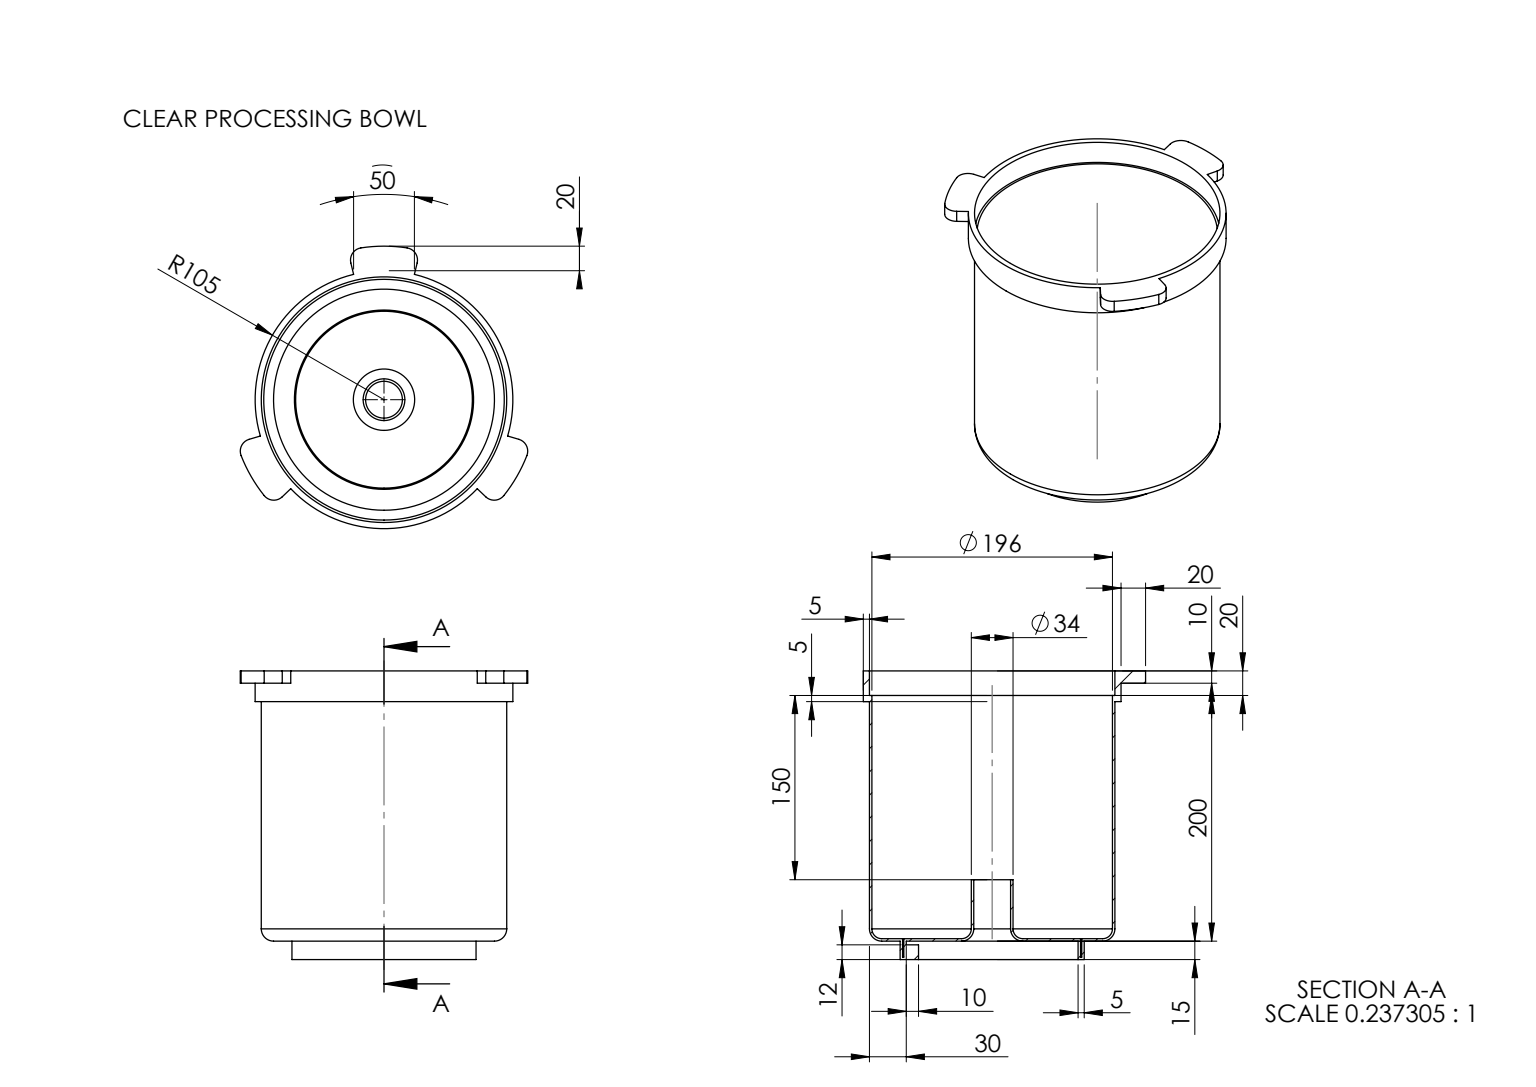
ISO-10303-21;
HEADER;
FILE_DESCRIPTION (('STEP AP214'),
    '1' );
FILE_NAME ('Clear Processing Bowl.step',
    '2026-10-08T14:59:03',
    ( '' ),
    ( '' ),
    'SwSTEP 2.0',
    'SolidWorks 2026',
    '' );
FILE_SCHEMA (( 'AUTOMOTIVE_DESIGN' ));
ENDSEC;

DATA;
#4=ORIENTED_EDGE ( 'NONE', *, *, #10707, .F. ) ;
#7=AXIS2_PLACEMENT_3D ( 'NONE', #9543, #8426, #7563 ) ;
#29=FACE_OUTER_BOUND ( 'NONE', #6935, .T. ) ;
#32=SURFACE_STYLE_FILL_AREA ( #12272 ) ;
#33=CARTESIAN_POINT ( 'NONE',  ( 0.000000000000000000, 62.00000000000000000, 0.000000000000000000 ) ) ;
#38=FACE_BOUND ( 'NONE', #4194, .T. ) ;
#43=CYLINDRICAL_SURFACE ( 'NONE', #5992, 70.00000000000001421 ) ;
#54=DIRECTION ( 'NONE',  ( -0.000000000000000000, -1.000000000000000000, -0.000000000000000000 ) ) ;
#56=ORIENTED_EDGE ( 'NONE', *, *, #12103, .T. ) ;
#69=AXIS2_PLACEMENT_3D ( 'NONE', #2443, #8100, #4365 ) ;
#71=CARTESIAN_POINT ( 'NONE',  ( 100.7495955565343593, 285.0000000000000568, 29.57226733266770680 ) ) ;
#83=EDGE_LOOP ( 'NONE', ( #1644, #11783, #306, #9102 ) ) ;
#85=DIRECTION ( 'NONE',  ( -0.000000000000000000, -1.000000000000000000, -0.000000000000000000 ) ) ;
#86=DIRECTION ( 'NONE',  ( 0.000000000000000000, 1.000000000000000000, 0.000000000000000000 ) ) ;
#87=CIRCLE ( 'NONE', #695, 73.00000000000002842 ) ;
#88=AXIS2_PLACEMENT_3D ( 'NONE', #4376, #577, #4254 ) ;
#89=EDGE_CURVE ( 'NONE', #9269, #3272, #10464, .T. ) ;
#92=ADVANCED_FACE ( 'NONE', ( #6517 ), #10949, .F. ) ;
#99=FACE_OUTER_BOUND ( 'NONE', #3781, .T. ) ;
#107=AXIS2_PLACEMENT_3D ( 'NONE', #11604, #10713, #5802 ) ;
#108=VERTEX_POINT ( 'NONE', #8368 ) ;
#109=CARTESIAN_POINT ( 'NONE',  ( 0.000000000000000000, 67.00000000000000000, -73.00000000000002842 ) ) ;
#113=DIRECTION ( 'NONE',  ( 0.000000000000000000, 1.000000000000000000, 0.000000000000000000 ) ) ;
#115=ORIENTED_EDGE ( 'NONE', *, *, #11098, .T. ) ;
#119=LINE ( 'NONE', #1007, #8979 ) ;
#120=DIRECTION ( 'NONE',  ( -0.2816406412635021894, 0.000000000000000000, 0.9595199576812789566 ) ) ;
#127=CARTESIAN_POINT ( 'NONE',  ( 89.80805993797383735, 285.0000000000000568, 71.82974571984303225 ) ) ;
#130=CARTESIAN_POINT ( 'NONE',  ( 1.836970198721029589E-15, 115.0000000000000142, 15.00000000000000000 ) ) ;
#145=ORIENTED_EDGE ( 'NONE', *, *, #5135, .F. ) ;
#146=CARTESIAN_POINT ( 'NONE',  ( -75.98513253586241945, 285.0000000000000568, 72.46557550663233371 ) ) ;
#147=CARTESIAN_POINT ( 'NONE',  ( 75.98513253586142469, 275.0000000000000000, 72.46557550663338532 ) ) ;
#152=AXIS2_PLACEMENT_3D ( 'NONE', #2615, #6425, #9273 ) ;
#154=EDGE_CURVE ( 'NONE', #8296, #4939, #9365, .T. ) ;
#165=ORIENTED_EDGE ( 'NONE', *, *, #7969, .F. ) ;
#166=CARTESIAN_POINT ( 'NONE',  ( 1.224646799147353533E-14, 265.0000000000000000, -100.0000000000000284 ) ) ;
#176=FACE_OUTER_BOUND ( 'NONE', #3457, .T. ) ;
#198=DIRECTION ( 'NONE',  ( -0.000000000000000000, -1.000000000000000000, 0.000000000000000000 ) ) ;
#216=AXIS2_PLACEMENT_3D ( 'NONE', #7014, #9871, #9743 ) ;
#223=VECTOR ( 'NONE', #5439, 1000.000000000000000 ) ;
#231=FACE_OUTER_BOUND ( 'NONE', #702, .T. ) ;
#233=ORIENTED_EDGE ( 'NONE', *, *, #10820, .F. ) ;
#235=ORIENTED_EDGE ( 'NONE', *, *, #9238, .T. ) ;
#238=ORIENTED_EDGE ( 'NONE', *, *, #5725, .T. ) ;
#244=DIRECTION ( 'NONE',  ( 0.000000000000000000, 0.000000000000000000, 1.000000000000000000 ) ) ;
#251=ORIENTED_EDGE ( 'NONE', *, *, #2932, .T. ) ;
#253=ADVANCED_FACE ( 'NONE', ( #8231 ), #12053, .T. ) ;
#256=CYLINDRICAL_SURFACE ( 'NONE', #8375, 105.0000000000000426 ) ;
#262=CIRCLE ( 'NONE', #10209, 75.00000000000002842 ) ;
#267=CIRCLE ( 'NONE', #8819, 105.0000000000000426 ) ;
#274=DIRECTION ( 'NONE',  ( 0.000000000000000000, 1.000000000000000000, 0.000000000000000000 ) ) ;
#285=CIRCLE ( 'NONE', #11657, 98.00000000000001421 ) ;
#299=CARTESIAN_POINT ( 'NONE',  ( 0.000000000000000000, 75.00000000000001421, 0.000000000000000000 ) ) ;
#306=ORIENTED_EDGE ( 'NONE', *, *, #8983, .F. ) ;
#318=ORIENTED_EDGE ( 'NONE', *, *, #11318, .F. ) ;
#342=FILL_AREA_STYLE ('',( #7079 ) ) ;
#356=STYLED_ITEM ( 'NONE', ( #4270 ), #8978 ) ;
#361=CARTESIAN_POINT ( 'NONE',  ( 6.000000000000000888, 62.00000000000000000, 60.00000000000002132 ) ) ;
#368=EDGE_CURVE ( 'NONE', #12219, #5612, #10551, .T. ) ;
#387=EDGE_LOOP ( 'NONE', ( #11646, #165 ) ) ;
#411=CYLINDRICAL_SURFACE ( 'NONE', #9069, 98.00000000000001421 ) ;
#413=TOROIDAL_SURFACE ( 'NONE', #613, 25.00000000000000000, 10.00000000000000000 ) ;
#417=ORIENTED_EDGE ( 'NONE', *, *, #6620, .F. ) ;
#419=AXIS2_PLACEMENT_3D ( 'NONE', #2678, #9277, #9505 ) ;
#424=DIRECTION ( 'NONE',  ( 0.000000000000000000, 1.000000000000000000, 0.000000000000000000 ) ) ;
#433=EDGE_CURVE ( 'NONE', #10879, #1577, #8550, .T. ) ;
#435=EDGE_CURVE ( 'NONE', #12106, #2099, #3183, .T. ) ;
#439=DIRECTION ( 'NONE',  ( 0.000000000000000000, 0.000000000000000000, -1.000000000000000000 ) ) ;
#440=PLANE ( 'NONE',  #3510 ) ;
#441=EDGE_LOOP ( 'NONE', ( #2108, #9208, #4543, #3626 ) ) ;
#453=ORIENTED_EDGE ( 'NONE', *, *, #3293, .T. ) ;
#456=AXIS2_PLACEMENT_3D ( 'NONE', #1243, #3050, #5051 ) ;
#460=FACE_OUTER_BOUND ( 'NONE', #3066, .T. ) ;
#461=MANIFOLD_SOLID_BREP ( 'Extrude-Thin3', #9257 ) ;
#465=AXIS2_PLACEMENT_3D ( 'NONE', #33, #11522, #7021 ) ;
#473=CIRCLE ( 'NONE', #5663, 90.00000000000002842 ) ;
#474=CIRCLE ( 'NONE', #4071, 8.000000000000007105 ) ;
#479=ORIENTED_EDGE ( 'NONE', *, *, #7943, .T. ) ;
#491=DIRECTION ( 'NONE',  ( 0.000000000000000000, 0.000000000000000000, 1.000000000000000000 ) ) ;
#492=DIRECTION ( 'NONE',  ( -0.000000000000000000, -1.000000000000000000, -0.000000000000000000 ) ) ;
#493=AXIS2_PLACEMENT_3D ( 'NONE', #11847, #424, #8951 ) ;
#502=DIRECTION ( 'NONE',  ( 0.000000000000000000, -1.000000000000000000, -0.000000000000000000 ) ) ;
#503=DIRECTION ( 'NONE',  ( -1.224646799147352961E-16, 0.000000000000000000, 1.000000000000000000 ) ) ;
#504=ORIENTED_EDGE ( 'NONE', *, *, #8965, .F. ) ;
#505=DIRECTION ( 'NONE',  ( 0.000000000000000000, 0.000000000000000000, -1.000000000000000000 ) ) ;
#507=CARTESIAN_POINT ( 'NONE',  ( 9.184850993605151889E-15, 65.00000000000000000, 75.00000000000002842 ) ) ;
#514=VECTOR ( 'NONE', #9075, 1000.000000000000000 ) ;
#516=CARTESIAN_POINT ( 'NONE',  ( -107.1104145097476987, 275.0000000000000000, 41.86118851095882576 ) ) ;
#519=CYLINDRICAL_SURFACE ( 'NONE', #3271, 98.00000000000001421 ) ;
#522=DIRECTION ( 'NONE',  ( 0.000000000000000000, 0.000000000000000000, 1.000000000000000000 ) ) ;
#523=CARTESIAN_POINT ( 'NONE',  ( 0.000000000000000000, 62.00000000000000000, 0.000000000000000000 ) ) ;
#524=DIRECTION ( 'NONE',  ( 0.000000000000000000, 0.000000000000000000, 1.000000000000000000 ) ) ;
#526=CIRCLE ( 'NONE', #5716, 73.00000000000002842 ) ;
#527=ADVANCED_FACE ( 'NONE', ( #2781 ), #9380, .T. ) ;
#544=VERTEX_POINT ( 'NONE', #4970 ) ;
#548=EDGE_CURVE ( 'NONE', #8705, #7192, #9752, .T. ) ;
#558=ORIENTED_EDGE ( 'NONE', *, *, #2494, .T. ) ;
#572=DIRECTION ( 'NONE',  ( 0.000000000000000000, 1.000000000000000000, 0.000000000000000000 ) ) ;
#577=DIRECTION ( 'NONE',  ( 0.000000000000000000, 1.000000000000000000, 0.000000000000000000 ) ) ;
#583=CARTESIAN_POINT ( 'NONE',  ( 18.80690714323171520, 275.0000000000000000, -123.5771024247852807 ) ) ;
#584=EDGE_CURVE ( 'NONE', #7474, #5986, #5098, .T. ) ;
#585=FACE_OUTER_BOUND ( 'NONE', #83, .T. ) ;
#594=LINE ( 'NONE', #10370, #1166 ) ;
#595=MECHANICAL_DESIGN_GEOMETRIC_PRESENTATION_REPRESENTATION('',(#5976),#2778);
#599=DIRECTION ( 'NONE',  ( 0.000000000000000000, 0.000000000000000000, 1.000000000000000000 ) ) ;
#603=FACE_OUTER_BOUND ( 'NONE', #4240, .T. ) ;
#612=AXIS2_PLACEMENT_3D ( 'NONE', #11738, #4009, #6752 ) ;
#613=AXIS2_PLACEMENT_3D ( 'NONE', #1971, #10567, #3032 ) ;
#617=DIRECTION ( 'NONE',  ( 0.000000000000000000, 0.000000000000000000, 1.000000000000000000 ) ) ;
#629=DIRECTION ( 'NONE',  ( 0.000000000000000000, 1.000000000000000000, 0.000000000000000000 ) ) ;
#631=AXIS2_PLACEMENT_3D ( 'NONE', #5538, #3719, #4470 ) ;
#633=DIRECTION ( 'NONE',  ( -0.000000000000000000, -1.000000000000000000, -0.000000000000000000 ) ) ;
#651=LINE ( 'NONE', #12127, #2432 ) ;
#654=CIRCLE ( 'NONE', #3836, 8.000000000000007105 ) ;
#659=CARTESIAN_POINT ( 'NONE',  ( 27.02024436599224444, 285.0000000000000568, -111.3324139431193203 ) ) ;
#662=FACE_BOUND ( 'NONE', #2461, .T. ) ;
#666=CARTESIAN_POINT ( 'NONE',  ( 1.151167991198512444E-14, 67.00000000000000000, -90.00000000000002842 ) ) ;
#672=DIRECTION ( 'NONE',  ( 0.000000000000000000, 1.000000000000000000, 0.000000000000000000 ) ) ;
#675=AXIS2_PLACEMENT_3D ( 'NONE', #3704, #10435, #7632 ) ;
#677=DIRECTION ( 'NONE',  ( 1.000000000000000000, 0.000000000000000000, 0.000000000000000000 ) ) ;
#679=CARTESIAN_POINT ( 'NONE',  ( 0.000000000000000000, 65.00000000000000000, 0.000000000000000000 ) ) ;
#693=VERTEX_POINT ( 'NONE', #659 ) ;
#695=AXIS2_PLACEMENT_3D ( 'NONE', #10958, #11786, #9012 ) ;
#699=CARTESIAN_POINT ( 'NONE',  ( -24.76446302067273209, 275.0000000000000000, -102.0378428393002679 ) ) ;
#702=EDGE_LOOP ( 'NONE', ( #8992, #2188, #4464, #4778, #1132, #2997, #10050, #6228, #2644, #12301, #5312, #7784, #1821, #3752, #12332, #4684, #6118, #9409, #9392, #3995, #6001 ) ) ;
#720=CARTESIAN_POINT ( 'NONE',  ( 0.000000000000000000, 75.00000000000001421, 0.000000000000000000 ) ) ;
#729=ADVANCED_FACE ( 'NONE', ( #6392 ), #9115, .T. ) ;
#731=DIRECTION ( 'NONE',  ( -1.000000000000000000, 0.000000000000000000, 0.000000000000000000 ) ) ;
#732=DIRECTION ( 'NONE',  ( 0.000000000000000000, 0.000000000000000000, 1.000000000000000000 ) ) ;
#733=CIRCLE ( 'NONE', #2527, 17.00000000000000000 ) ;
#744=CARTESIAN_POINT ( 'NONE',  ( 0.000000000000000000, 75.00000000000001421, 0.000000000000000000 ) ) ;
#745=CARTESIAN_POINT ( 'NONE',  ( 0.000000000000000000, 275.0000000000000000, 0.000000000000000000 ) ) ;
#761=EDGE_CURVE ( 'NONE', #10706, #2323, #7254, .T. ) ;
#765=DIRECTION ( 'NONE',  ( 0.000000000000000000, 0.000000000000000000, -1.000000000000000000 ) ) ;
#770=EDGE_CURVE ( 'NONE', #5668, #544, #8820, .T. ) ;
#786=DIRECTION ( 'NONE',  ( 0.6901483381584130328, 0.000000000000000000, -0.7236679289129654968 ) ) ;
#791=CIRCLE ( 'NONE', #10362, 10.00000000000000178 ) ;
#793=DIRECTION ( 'NONE',  ( 0.2816406412634883671, -0.000000000000000000, 0.9595199576812829534 ) ) ;
#803=LINE ( 'NONE', #5605, #6040 ) ;
#830=CARTESIAN_POINT ( 'NONE',  ( 0.000000000000000000, 75.00000000000001421, 0.000000000000000000 ) ) ;
#851=ORIENTED_EDGE ( 'NONE', *, *, #11796, .T. ) ;
#860=CARTESIAN_POINT ( 'NONE',  ( 0.000000000000000000, 62.00000000000000000, 0.000000000000000000 ) ) ;
#874=CIRCLE ( 'NONE', #11828, 75.00000000000002842 ) ;
#886=ORIENTED_EDGE ( 'NONE', *, *, #12003, .F. ) ;
#894=AXIS2_PLACEMENT_3D ( 'NONE', #1113, #1048, #3976 ) ;
#901=EDGE_CURVE ( 'NONE', #7094, #2243, #9622, .T. ) ;
#906=ORIENTED_EDGE ( 'NONE', *, *, #548, .F. ) ;
#907=AXIS2_PLACEMENT_3D ( 'NONE', #8234, #11997, #1392 ) ;
#911=DIRECTION ( 'NONE',  ( 0.000000000000000000, 1.000000000000000000, 0.000000000000000000 ) ) ;
#926=EDGE_CURVE ( 'NONE', #6039, #4819, #473, .T. ) ;
#939=LINE ( 'NONE', #8710, #3742 ) ;
#943=DIRECTION ( 'NONE',  ( 0.000000000000000000, 0.000000000000000000, 1.000000000000000000 ) ) ;
#950=VERTEX_POINT ( 'NONE', #2146 ) ;
#978=DIRECTION ( 'NONE',  ( 0.000000000000000000, -1.000000000000000000, 0.000000000000000000 ) ) ;
#990=DIRECTION ( 'NONE',  ( -0.5000000000000012212, 0.000000000000000000, -0.8660254037844379305 ) ) ;
#991=LINE ( 'NONE', #4979, #7553 ) ;
#992=AXIS2_PLACEMENT_3D ( 'NONE', #10845, #4177, #11674 ) ;
#1001=DIRECTION ( 'NONE',  ( 0.000000000000000000, 0.000000000000000000, 1.000000000000000000 ) ) ;
#1007=CARTESIAN_POINT ( 'NONE',  ( 0.000000000000000000, 265.0000000000000000, -98.00000000000001421 ) ) ;
#1008=PLANE ( 'NONE',  #3807 ) ;
#1023=CARTESIAN_POINT ( 'NONE',  ( 0.000000000000000000, 75.00000000000001421, 0.000000000000000000 ) ) ;
#1034=CARTESIAN_POINT ( 'NONE',  ( 0.000000000000000000, 265.0000000000000000, 0.000000000000000000 ) ) ;
#1036=LINE ( 'NONE', #3773, #6303 ) ;
#1048=DIRECTION ( 'NONE',  ( 0.000000000000000000, 1.000000000000000000, 0.000000000000000000 ) ) ;
#1055=VECTOR ( 'NONE', #1123, 1000.000000000000000 ) ;
#1064=CARTESIAN_POINT ( 'NONE',  ( 2.081899558550500280E-15, 265.0000000000000000, 17.00000000000000000 ) ) ;
#1067=ORIENTED_EDGE ( 'NONE', *, *, #6888, .T. ) ;
#1082=PLANE ( 'NONE',  #10248 ) ;
#1083=CARTESIAN_POINT ( 'NONE',  ( -75.98513253586240523, 275.0000000000000000, 72.46557550663233371 ) ) ;
#1090=AXIS2_PLACEMENT_3D ( 'NONE', #8302, #9230, #3328 ) ;
#1093=DIRECTION ( 'NONE',  ( 0.000000000000000000, 0.000000000000000000, 1.000000000000000000 ) ) ;
#1105=ADVANCED_FACE ( 'NONE', ( #11058 ), #8235, .T. ) ;
#1113=CARTESIAN_POINT ( 'NONE',  ( 0.000000000000000000, 285.0000000000000568, 0.000000000000000000 ) ) ;
#1117=ORIENTED_EDGE ( 'NONE', *, *, #9037, .T. ) ;
#1121=ADVANCED_FACE ( 'NONE', ( #5205 ), #519, .F. ) ;
#1123=DIRECTION ( 'NONE',  ( 0.000000000000000000, 1.000000000000000000, 0.000000000000000000 ) ) ;
#1125=ADVANCED_FACE ( 'NONE', ( #8177, #12124 ), #9103, .F. ) ;
#1126=CARTESIAN_POINT ( 'NONE',  ( 0.000000000000000000, 75.00000000000001421, 0.000000000000000000 ) ) ;
#1127=CARTESIAN_POINT ( 'NONE',  ( 90.45849111412074706, 285.0000000000000568, 86.26854226980164242 ) ) ;
#1132=ORIENTED_EDGE ( 'NONE', *, *, #7766, .T. ) ;
#1137=EDGE_CURVE ( 'NONE', #7815, #2386, #7462, .T. ) ;
#1147=CYLINDRICAL_SURFACE ( 'NONE', #7579, 70.00000000000001421 ) ;
#1148=DIRECTION ( 'NONE',  ( 0.000000000000000000, 0.000000000000000000, 1.000000000000000000 ) ) ;
#1157=DIRECTION ( 'NONE',  ( 0.000000000000000000, 1.000000000000000000, 0.000000000000000000 ) ) ;
#1158=FACE_OUTER_BOUND ( 'NONE', #10972, .T. ) ;
#1162=CIRCLE ( 'NONE', #9701, 10.00000000000000178 ) ;
#1166=VECTOR ( 'NONE', #6523, 1000.000000000000227 ) ;
#1167=DIRECTION ( 'NONE',  ( 0.000000000000000000, 1.000000000000000000, 0.000000000000000000 ) ) ;
#1172=DIRECTION ( 'NONE',  ( -0.000000000000000000, -1.000000000000000000, -0.000000000000000000 ) ) ;
#1178=DIRECTION ( 'NONE',  ( -0.000000000000000000, -1.000000000000000000, 0.000000000000000000 ) ) ;
#1187=PLANE ( 'NONE',  #3304 ) ;
#1206=VECTOR ( 'NONE', #6312, 1000.000000000000000 ) ;
#1213=VECTOR ( 'NONE', #5291, 1000.000000000000000 ) ;
#1226=VECTOR ( 'NONE', #7740, 1000.000000000000000 ) ;
#1232=DIRECTION ( 'NONE',  ( 0.000000000000000000, 0.000000000000000000, 1.000000000000000000 ) ) ;
#1243=CARTESIAN_POINT ( 'NONE',  ( 29.48150359603894088, 275.0000000000000000, -121.4736224277384053 ) ) ;
#1247=EDGE_LOOP ( 'NONE', ( #4101, #9105, #8582, #1067 ) ) ;
#1254=CIRCLE ( 'NONE', #10203, 100.0000000000000142 ) ;
#1258=DIRECTION ( 'NONE',  ( 1.000000000000000000, 0.000000000000000000, 0.000000000000000000 ) ) ;
#1261=CARTESIAN_POINT ( 'NONE',  ( -24.76446302067273209, 275.0000000000000000, -102.0378428393002679 ) ) ;
#1266=CIRCLE ( 'NONE', #8214, 100.0000000000000284 ) ;
#1268=DIRECTION ( 'NONE',  ( -0.000000000000000000, -1.000000000000000000, -0.000000000000000000 ) ) ;
#1271=CYLINDRICAL_SURFACE ( 'NONE', #5282, 10.00000000000000178 ) ;
#1275=PRODUCT_DEFINITION_CONTEXT ( 'detailed design', #10350, 'design' ) ;
#1278=VERTEX_POINT ( 'NONE', #2755 ) ;
#1280=CARTESIAN_POINT ( 'NONE',  ( -100.7495955565347288, 275.0000000000000000, 29.57226733266632124 ) ) ;
#1286=ORIENTED_EDGE ( 'NONE', *, *, #1936, .F. ) ;
#1326=LINE ( 'NONE', #8101, #11490 ) ;
#1332=VECTOR ( 'NONE', #9870, 1000.000000000000227 ) ;
#1335=FACE_BOUND ( 'NONE', #4548, .T. ) ;
#1337=ORIENTED_EDGE ( 'NONE', *, *, #10508, .F. ) ;
#1338=DIRECTION ( 'NONE',  ( 0.000000000000000000, 1.000000000000000000, 0.000000000000000000 ) ) ;
#1342=VECTOR ( 'NONE', #10158, 1000.000000000000114 ) ;
#1343=CARTESIAN_POINT ( 'NONE',  ( 0.000000000000000000, 67.00000000000000000, 0.000000000000000000 ) ) ;
#1358=ADVANCED_FACE ( 'NONE', ( #5003 ), #256, .T. ) ;
#1360=( GEOMETRIC_REPRESENTATION_CONTEXT ( 3 ) GLOBAL_UNCERTAINTY_ASSIGNED_CONTEXT ( ( #9114 ) ) GLOBAL_UNIT_ASSIGNED_CONTEXT ( ( #3339, #10754, #4149 ) ) REPRESENTATION_CONTEXT ( 'NONE', 'WORKASPACE' ) );
#1392=DIRECTION ( 'NONE',  ( 0.000000000000000000, 0.000000000000000000, 1.000000000000000000 ) ) ;
#1405=EDGE_LOOP ( 'NONE', ( #115, #8358 ) ) ;
#1408=VECTOR ( 'NONE', #8580, 1000.000000000000000 ) ;
#1429=VERTEX_POINT ( 'NONE', #5998 ) ;
#1430=AXIS2_PLACEMENT_3D ( 'NONE', #10005, #3409, #12081 ) ;
#1435=DIRECTION ( 'NONE',  ( -0.000000000000000000, -1.000000000000000000, -0.000000000000000000 ) ) ;
#1437=CARTESIAN_POINT ( 'NONE',  ( 0.000000000000000000, 67.00000000000000000, 0.000000000000000000 ) ) ;
#1438=VERTEX_POINT ( 'NONE', #130 ) ;
#1440=CARTESIAN_POINT ( 'NONE',  ( 0.000000000000000000, 75.00000000000001421, 0.000000000000000000 ) ) ;
#1441=EDGE_CURVE ( 'NONE', #7734, #7317, #3067, .T. ) ;
#1446=ADVANCED_FACE ( 'NONE', ( #6811 ), #2071, .T. ) ;
#1456=EDGE_CURVE ( 'NONE', #2323, #9195, #9966, .T. ) ;
#1469=SURFACE_STYLE_USAGE ( .BOTH. , #10878 ) ;
#1473=DIRECTION ( 'NONE',  ( 0.000000000000000000, -1.000000000000000000, 0.000000000000000000 ) ) ;
#1477=FACE_OUTER_BOUND ( 'NONE', #4787, .T. ) ;
#1490=ORIENTED_EDGE ( 'NONE', *, *, #5036, .F. ) ;
#1494=VECTOR ( 'NONE', #6669, 1000.000000000000000 ) ;
#1500=VERTEX_POINT ( 'NONE', #6365 ) ;
#1507=DIRECTION ( 'NONE',  ( -1.000000000000000000, 0.000000000000000000, -1.224646799147352961E-16 ) ) ;
#1518=VERTEX_POINT ( 'NONE', #9150 ) ;
#1525=ORIENTED_EDGE ( 'NONE', *, *, #2688, .T. ) ;
#1526=DIRECTION ( 'NONE',  ( 0.000000000000000000, 1.000000000000000000, 0.000000000000000000 ) ) ;
#1529=VECTOR ( 'NONE', #7637, 1000.000000000000000 ) ;
#1535=CIRCLE ( 'NONE', #2530, 17.00000000000000000 ) ;
#1541=DIRECTION ( 'NONE',  ( 0.000000000000000000, 0.000000000000000000, 1.000000000000000000 ) ) ;
#1542=PLANE ( 'NONE',  #3430 ) ;
#1577=VERTEX_POINT ( 'NONE', #6242 ) ;
#1580=ORIENTED_EDGE ( 'NONE', *, *, #6196, .T. ) ;
#1595=EDGE_CURVE ( 'NONE', #2259, #7474, #11789, .T. ) ;
#1597=FACE_OUTER_BOUND ( 'NONE', #1247, .T. ) ;
#1612=AXIS2_PLACEMENT_3D ( 'NONE', #9562, #7823, #5032 ) ;
#1615=DIRECTION ( 'NONE',  ( 0.000000000000000000, -1.000000000000000000, 0.000000000000000000 ) ) ;
#1620=CARTESIAN_POINT ( 'NONE',  ( 0.000000000000000000, 285.0000000000000568, 0.000000000000000000 ) ) ;
#1628=EDGE_LOOP ( 'NONE', ( #11303, #10262, #5115, #4111 ) ) ;
#1638=DIRECTION ( 'NONE',  ( 0.000000000000000000, 0.000000000000000000, -1.000000000000000000 ) ) ;
#1644=ORIENTED_EDGE ( 'NONE', *, *, #9873, .F. ) ;
#1649=CARTESIAN_POINT ( 'NONE',  ( -109.9268209223825750, 275.0000000000000000, 32.26598893414599445 ) ) ;
#1658=DIRECTION ( 'NONE',  ( 0.000000000000000000, 0.000000000000000000, 1.000000000000000000 ) ) ;
#1662=LINE ( 'NONE', #9559, #1529 ) ;
#1665=VECTOR ( 'NONE', #6592, 1000.000000000000000 ) ;
#1674=FACE_OUTER_BOUND ( 'NONE', #6355, .T. ) ;
#1681=ADVANCED_FACE ( 'NONE', ( #3971 ), #8284, .F. ) ;
#1711=ADVANCED_FACE ( 'NONE', ( #11229 ), #8633, .T. ) ;
#1724=DIRECTION ( 'NONE',  ( 0.000000000000000000, 0.000000000000000000, 1.000000000000000000 ) ) ;
#1725=CIRCLE ( 'NONE', #9672, 9.999999999999994671 ) ;
#1735=CARTESIAN_POINT ( 'NONE',  ( -119.9399947101603772, 285.0000000000000568, 35.20508015793608081 ) ) ;
#1738=ORIENTED_EDGE ( 'NONE', *, *, #11532, .F. ) ;
#1742=ORIENTED_EDGE ( 'NONE', *, *, #2513, .T. ) ;
#1744=VERTEX_POINT ( 'NONE', #8698 ) ;
#1755=CARTESIAN_POINT ( 'NONE',  ( -82.90657655639077461, 275.0000000000000000, 79.06642500897154946 ) ) ;
#1780=VECTOR ( 'NONE', #2713, 1000.000000000000000 ) ;
#1781=CARTESIAN_POINT ( 'NONE',  ( 0.000000000000000000, 52.00000000000000711, 0.000000000000000000 ) ) ;
#1789=ORIENTED_EDGE ( 'NONE', *, *, #7766, .F. ) ;
#1800=CIRCLE ( 'NONE', #4387, 98.00000000000001421 ) ;
#1801=CIRCLE ( 'NONE', #11565, 9.999999999999994671 ) ;
#1803=ORIENTED_EDGE ( 'NONE', *, *, #4104, .F. ) ;
#1816=EDGE_LOOP ( 'NONE', ( #6729, #7569, #2705, #7619 ) ) ;
#1821=ORIENTED_EDGE ( 'NONE', *, *, #2734, .T. ) ;
#1838=AXIS2_PLACEMENT_3D ( 'NONE', #3085, #6891, #522 ) ;
#1839=ORIENTED_EDGE ( 'NONE', *, *, #9686, .T. ) ;
#1841=CARTESIAN_POINT ( 'NONE',  ( 0.000000000000000000, 265.0000000000000000, 0.000000000000000000 ) ) ;
#1849=ORIENTED_EDGE ( 'NONE', *, *, #8354, .T. ) ;
#1851=CARTESIAN_POINT ( 'NONE',  ( 0.000000000000000000, 285.0000000000000568, 105.0000000000000426 ) ) ;
#1869=CYLINDRICAL_SURFACE ( 'NONE', #4026, 9.999999999999994671 ) ;
#1878=ORIENTED_EDGE ( 'NONE', *, *, #10963, .T. ) ;
#1884=CARTESIAN_POINT ( 'NONE',  ( 0.000000000000000000, 265.0000000000000000, 0.000000000000000000 ) ) ;
#1894=TOROIDAL_SURFACE ( 'NONE', #8255, 90.00000000000002842, 8.000000000000000000 ) ;
#1898=AXIS2_PLACEMENT_3D ( 'NONE', #860, #4654, #3720 ) ;
#1909=CIRCLE ( 'NONE', #8861, 10.00000000000000178 ) ;
#1919=FACE_OUTER_BOUND ( 'NONE', #3235, .T. ) ;
#1935=ORIENTED_EDGE ( 'NONE', *, *, #9515, .T. ) ;
#1936=EDGE_CURVE ( 'NONE', #5710, #7852, #2422, .T. ) ;
#1944=ORIENTED_EDGE ( 'NONE', *, *, #12194, .T. ) ;
#1952=CARTESIAN_POINT ( 'NONE',  ( 0.000000000000000000, 65.00000000000000000, 0.000000000000000000 ) ) ;
#1964=EDGE_CURVE ( 'NONE', #5986, #7898, #10984, .T. ) ;
#1971=CARTESIAN_POINT ( 'NONE',  ( 0.000000000000000000, 75.00000000000001421, 0.000000000000000000 ) ) ;
#1973=ADVANCED_FACE ( 'NONE', ( #1597 ), #7398, .T. ) ;
#1982=CIRCLE ( 'NONE', #2777, 10.00000000000000178 ) ;
#1987=ADVANCED_FACE ( 'NONE', ( #9119 ), #11951, .T. ) ;
#1988=ADVANCED_FACE ( 'NONE', ( #2650 ), #5616, .F. ) ;
#1993=LINE ( 'NONE', #9706, #1494 ) ;
#1995=VERTEX_POINT ( 'NONE', #6273 ) ;
#1997=CARTESIAN_POINT ( 'NONE',  ( 0.000000000000000000, 65.00000000000000000, -70.00000000000001421 ) ) ;
#2007=CARTESIAN_POINT ( 'NONE',  ( -89.80805993797480369, 285.0000000000000568, 81.82974571984181011 ) ) ;
#2014=DIRECTION ( 'NONE',  ( 0.000000000000000000, -0.000000000000000000, 1.000000000000000000 ) ) ;
#2032=CIRCLE ( 'NONE', #9579, 9.999999999999994671 ) ;
#2036=ADVANCED_FACE ( 'NONE', ( #8130 ), #5531, .F. ) ;
#2037=ADVANCED_FACE ( 'NONE', ( #9184, #662 ), #8377, .T. ) ;
#2054=CARTESIAN_POINT ( 'NONE',  ( 0.000000000000000000, 260.0000000000000000, 105.0000000000000426 ) ) ;
#2062=EDGE_CURVE ( 'NONE', #4939, #2386, #791, .T. ) ;
#2065=VECTOR ( 'NONE', #5965, 1000.000000000000114 ) ;
#2071=CYLINDRICAL_SURFACE ( 'NONE', #7788, 9.999999999999994671 ) ;
#2083=AXIS2_PLACEMENT_3D ( 'NONE', #3919, #8638, #990 ) ;
#2091=CARTESIAN_POINT ( 'NONE',  ( -89.80805993797480369, 275.0000000000000000, 71.82974571984181011 ) ) ;
#2096=ORIENTED_EDGE ( 'NONE', *, *, #11598, .F. ) ;
#2099=VERTEX_POINT ( 'NONE', #9372 ) ;
#2104=DIRECTION ( 'NONE',  ( 0.000000000000000000, 1.000000000000000000, 0.000000000000000000 ) ) ;
#2108=ORIENTED_EDGE ( 'NONE', *, *, #7108, .F. ) ;
#2115=AXIS2_PLACEMENT_3D ( 'NONE', #745, #1615, #6476 ) ;
#2129=CIRCLE ( 'NONE', #9484, 125.0000000000000284 ) ;
#2130=ORIENTED_EDGE ( 'NONE', *, *, #1964, .T. ) ;
#2146=CARTESIAN_POINT ( 'NONE',  ( 0.000000000000000000, 265.0000000000000000, 100.0000000000000284 ) ) ;
#2152=DIRECTION ( 'NONE',  ( 0.000000000000000000, 0.000000000000000000, -1.000000000000000000 ) ) ;
#2156=EDGE_CURVE ( 'NONE', #7734, #4551, #8738, .T. ) ;
#2159=CARTESIAN_POINT ( 'NONE',  ( -6.000000000000000000, 62.00000000000000000, 70.00000000000001421 ) ) ;
#2160=AXIS2_PLACEMENT_3D ( 'NONE', #8559, #9307, #9427 ) ;
#2161=DIRECTION ( 'NONE',  ( 0.000000000000000000, 0.000000000000000000, 1.000000000000000000 ) ) ;
#2166=DIRECTION ( 'NONE',  ( 0.000000000000000000, 1.000000000000000000, 0.000000000000000000 ) ) ;
#2168=ORIENTED_EDGE ( 'NONE', *, *, #1456, .T. ) ;
#2169=CARTESIAN_POINT ( 'NONE',  ( 0.000000000000000000, 275.0000000000000000, 0.000000000000000000 ) ) ;
#2177=CARTESIAN_POINT ( 'NONE',  ( 9.184850993605151889E-15, 50.00000000000000000, 75.00000000000002842 ) ) ;
#2178=ORIENTED_EDGE ( 'NONE', *, *, #2305, .T. ) ;
#2188=ORIENTED_EDGE ( 'NONE', *, *, #1595, .T. ) ;
#2207=LINE ( 'NONE', #6016, #11478 ) ;
#2210=CARTESIAN_POINT ( 'NONE',  ( 0.000000000000000000, 67.00000000000000000, 25.00000000000000000 ) ) ;
#2214=ADVANCED_FACE ( 'NONE', ( #8625 ), #4646, .T. ) ;
#2228=ORIENTED_EDGE ( 'NONE', *, *, #8855, .T. ) ;
#2238=CARTESIAN_POINT ( 'NONE',  ( 8.939921633775681592E-15, 65.00000000000000000, 73.00000000000002842 ) ) ;
#2239=EDGE_CURVE ( 'NONE', #11257, #4695, #6763, .T. ) ;
#2243=VERTEX_POINT ( 'NONE', #6526 ) ;
#2244=DIRECTION ( 'NONE',  ( 0.000000000000000000, 0.000000000000000000, 1.000000000000000000 ) ) ;
#2249=EDGE_CURVE ( 'NONE', #5904, #9892, #8139, .T. ) ;
#2257=ADVANCED_FACE ( 'NONE', ( #10374 ), #2772, .T. ) ;
#2259=VERTEX_POINT ( 'NONE', #4961 ) ;
#2270=DIRECTION ( 'NONE',  ( -0.000000000000000000, -1.000000000000000000, -0.000000000000000000 ) ) ;
#2286=DIRECTION ( 'NONE',  ( -0.7236679289129753778, 0.000000000000000000, 0.6901483381584025967 ) ) ;
#2287=CARTESIAN_POINT ( 'NONE',  ( -116.4243635975518742, 275.0000000000000000, 45.50129185973785440 ) ) ;
#2291=EDGE_CURVE ( 'NONE', #12245, #5612, #7386, .T. ) ;
#2292=VECTOR ( 'NONE', #1172, 1000.000000000000000 ) ;
#2293=CIRCLE ( 'NONE', #69, 90.00000000000002842 ) ;
#2305=EDGE_CURVE ( 'NONE', #4827, #12106, #9680, .T. ) ;
#2314=FACE_BOUND ( 'NONE', #10934, .T. ) ;
#2323=VERTEX_POINT ( 'NONE', #3265 ) ;
#2334=ADVANCED_FACE ( 'NONE', ( #4084, #1158 ), #4024, .F. ) ;
#2348=CARTESIAN_POINT ( 'NONE',  ( 1.285879139104721264E-14, 260.0000000000000000, -105.0000000000000426 ) ) ;
#2361=VERTEX_POINT ( 'NONE', #2210 ) ;
#2368=AXIS2_PLACEMENT_3D ( 'NONE', #8807, #274, #7012 ) ;
#2376=VERTEX_POINT ( 'NONE', #3333 ) ;
#2382=FACE_OUTER_BOUND ( 'NONE', #8509, .T. ) ;
#2386=VERTEX_POINT ( 'NONE', #9992 ) ;
#2391=CARTESIAN_POINT ( 'NONE',  ( 0.000000000000000000, 260.0000000000000000, 0.000000000000000000 ) ) ;
#2395=AXIS2_PLACEMENT_3D ( 'NONE', #8079, #11840, #8888 ) ;
#2405=AXIS2_PLACEMENT_3D ( 'NONE', #10012, #786, #2410 ) ;
#2406=LINE ( 'NONE', #6338, #5017 ) ;
#2409=EDGE_CURVE ( 'NONE', #8944, #2376, #10932, .T. ) ;
#2410=DIRECTION ( 'NONE',  ( -0.7236679289129653858, 0.000000000000000000, -0.6901483381584129218 ) ) ;
#2415=AXIS2_PLACEMENT_3D ( 'NONE', #6801, #9651, #244 ) ;
#2422=CIRCLE ( 'NONE', #1430, 105.0000000000000284 ) ;
#2432=VECTOR ( 'NONE', #3576, 1000.000000000000000 ) ;
#2436=VERTEX_POINT ( 'NONE', #7439 ) ;
#2443=CARTESIAN_POINT ( 'NONE',  ( 0.000000000000000000, 65.00000000000000000, 0.000000000000000000 ) ) ;
#2448=CIRCLE ( 'NONE', #11625, 9.999999999999994671 ) ;
#2452=CYLINDRICAL_SURFACE ( 'NONE', #907, 100.0000000000000284 ) ;
#2454=CARTESIAN_POINT ( 'NONE',  ( 0.000000000000000000, 65.00000000000000000, 0.000000000000000000 ) ) ;
#2456=VECTOR ( 'NONE', #3663, 1000.000000000000000 ) ;
#2461=EDGE_LOOP ( 'NONE', ( #4068, #8388 ) ) ;
#2464=AXIS2_PLACEMENT_3D ( 'NONE', #11019, #8892, #11905 ) ;
#2472=CARTESIAN_POINT ( 'NONE',  ( 0.000000000000000000, 67.00000000000000000, 90.00000000000002842 ) ) ;
#2485=DIRECTION ( 'NONE',  ( -0.000000000000000000, -1.000000000000000000, -0.000000000000000000 ) ) ;
#2489=CARTESIAN_POINT ( 'NONE',  ( 1.224646799147353375E-14, 265.0000000000000000, 100.0000000000000142 ) ) ;
#2491=ORIENTED_EDGE ( 'NONE', *, *, #7520, .T. ) ;
#2494=EDGE_CURVE ( 'NONE', #12345, #5565, #3580, .T. ) ;
#2497=DIRECTION ( 'NONE',  ( 0.000000000000000000, 1.000000000000000000, 0.000000000000000000 ) ) ;
#2501=DIRECTION ( 'NONE',  ( 0.000000000000000000, 0.000000000000000000, 1.000000000000000000 ) ) ;
#2513=EDGE_CURVE ( 'NONE', #2361, #6532, #8342, .T. ) ;
#2515=ORIENTED_EDGE ( 'NONE', *, *, #8242, .F. ) ;
#2527=AXIS2_PLACEMENT_3D ( 'NONE', #11326, #2773, #5408 ) ;
#2530=AXIS2_PLACEMENT_3D ( 'NONE', #720, #12128, #3637 ) ;
#2533=CARTESIAN_POINT ( 'NONE',  ( 0.000000000000000000, 75.00000000000001421, 0.000000000000000000 ) ) ;
#2554=VERTEX_POINT ( 'NONE', #2571 ) ;
#2566=LINE ( 'NONE', #9222, #9544 ) ;
#2570=ORIENTED_EDGE ( 'NONE', *, *, #9023, .F. ) ;
#2571=CARTESIAN_POINT ( 'NONE',  ( 100.7495955565343451, 275.0000000000000000, 29.57226733266770680 ) ) ;
#2577=CARTESIAN_POINT ( 'NONE',  ( 0.000000000000000000, 65.00000000000000000, 0.000000000000000000 ) ) ;
#2580=VECTOR ( 'NONE', #5484, 1000.000000000000000 ) ;
#2581=AXIS2_PLACEMENT_3D ( 'NONE', #2633, #8233, #12057 ) ;
#2590=DIRECTION ( 'NONE',  ( 0.000000000000000000, 1.000000000000000000, 0.000000000000000000 ) ) ;
#2592=PLANE ( 'NONE',  #10054 ) ;
#2599=AXIS2_PLACEMENT_3D ( 'NONE', #2169, #7656, #10462 ) ;
#2602=VERTEX_POINT ( 'NONE', #2007 ) ;
#2604=LINE ( 'NONE', #1735, #8619 ) ;
#2615=CARTESIAN_POINT ( 'NONE',  ( 0.000000000000000000, 285.0000000000000568, 0.000000000000000000 ) ) ;
#2633=CARTESIAN_POINT ( 'NONE',  ( 0.000000000000000000, 65.00000000000000000, 0.000000000000000000 ) ) ;
#2639=DIRECTION ( 'NONE',  ( 1.000000000000000000, 0.000000000000000000, -1.065814103640150437E-14 ) ) ;
#2644=ORIENTED_EDGE ( 'NONE', *, *, #8199, .F. ) ;
#2650=FACE_OUTER_BOUND ( 'NONE', #8310, .T. ) ;
#2658=EDGE_CURVE ( 'NONE', #4082, #5298, #12340, .T. ) ;
#2661=LINE ( 'NONE', #6473, #1665 ) ;
#2667=CARTESIAN_POINT ( 'NONE',  ( 1.200153863164406345E-14, 75.00000000000001421, 98.00000000000001421 ) ) ;
#2670=DIRECTION ( 'NONE',  ( 0.000000000000000000, 1.000000000000000000, 0.000000000000000000 ) ) ;
#2671=AXIS2_PLACEMENT_3D ( 'NONE', #2454, #6195, #8986 ) ;
#2673=ORIENTED_EDGE ( 'NONE', *, *, #5949, .F. ) ;
#2677=ORIENTED_EDGE ( 'NONE', *, *, #11274, .T. ) ;
#2678=CARTESIAN_POINT ( 'NONE',  ( -17.30235457177319347, 275.0000000000000000, -113.6909342308024549 ) ) ;
#2688=EDGE_CURVE ( 'NONE', #544, #5668, #5175, .T. ) ;
#2694=CARTESIAN_POINT ( 'NONE',  ( 0.000000000000000000, 67.00000000000000000, 0.000000000000000000 ) ) ;
#2700=CARTESIAN_POINT ( 'NONE',  ( -17.30235457177319347, 285.0000000000000568, -113.6909342308024549 ) ) ;
#2705=ORIENTED_EDGE ( 'NONE', *, *, #7052, .T. ) ;
#2713=DIRECTION ( 'NONE',  ( 0.000000000000000000, 1.000000000000000000, 0.000000000000000000 ) ) ;
#2714=AXIS2_PLACEMENT_3D ( 'NONE', #2391, #7879, #524 ) ;
#2732=EDGE_CURVE ( 'NONE', #3744, #2602, #4767, .T. ) ;
#2734=EDGE_CURVE ( 'NONE', #3401, #4827, #6363, .T. ) ;
#2755=CARTESIAN_POINT ( 'NONE',  ( 0.000000000000000000, 285.0000000000000568, 100.0000000000000284 ) ) ;
#2772=CYLINDRICAL_SURFACE ( 'NONE', #10557, 9.999999999999994671 ) ;
#2773=DIRECTION ( 'NONE',  ( 0.000000000000000000, 1.000000000000000000, 0.000000000000000000 ) ) ;
#2776=DIRECTION ( 'NONE',  ( 0.5000000000000039968, 0.000000000000000000, -0.8660254037844363761 ) ) ;
#2777=AXIS2_PLACEMENT_3D ( 'NONE', #11528, #1178, #4920 ) ;
#2778=( GEOMETRIC_REPRESENTATION_CONTEXT ( 3 ) GLOBAL_UNCERTAINTY_ASSIGNED_CONTEXT ( ( #5276 ) ) GLOBAL_UNIT_ASSIGNED_CONTEXT ( ( #5723, #4777, #10510 ) ) REPRESENTATION_CONTEXT ( 'NONE', 'WORKASPACE' ) );
#2781=FACE_OUTER_BOUND ( 'NONE', #6057, .T. ) ;
#2789=CARTESIAN_POINT ( 'NONE',  ( 8.939921633775681592E-15, 52.00000000000000711, 73.00000000000002842 ) ) ;
#2796=AXIS2_PLACEMENT_3D ( 'NONE', #9436, #4652, #2776 ) ;
#2797=AXIS2_PLACEMENT_3D ( 'NONE', #1841, #85, #2838 ) ;
#2802=CARTESIAN_POINT ( 'NONE',  ( 0.000000000000000000, 65.00000000000000000, -70.00000000000001421 ) ) ;
#2816=VERTEX_POINT ( 'NONE', #8963 ) ;
#2818=DIRECTION ( 'NONE',  ( 0.000000000000000000, 1.000000000000000000, 0.000000000000000000 ) ) ;
#2829=CARTESIAN_POINT ( 'NONE',  ( 0.000000000000000000, 67.00000000000000000, 0.000000000000000000 ) ) ;
#2838=DIRECTION ( 'NONE',  ( 0.000000000000000000, 0.000000000000000000, -1.000000000000000000 ) ) ;
#2851=DIRECTION ( 'NONE',  ( 0.000000000000000000, 1.000000000000000000, 0.000000000000000000 ) ) ;
#2865=EDGE_LOOP ( 'NONE', ( #7611, #6742, #1849, #9784, #12183, #7498, #56, #6864, #6783, #318 ) ) ;
#2867=FACE_OUTER_BOUND ( 'NONE', #8250, .T. ) ;
#2870=AXIS2_PLACEMENT_3D ( 'NONE', #6382, #7190, #10992 ) ;
#2875=EDGE_CURVE ( 'NONE', #4551, #4695, #8510, .T. ) ;
#2891=ORIENTED_EDGE ( 'NONE', *, *, #11765, .T. ) ;
#2900=FACE_BOUND ( 'NONE', #8062, .T. ) ;
#2905=VECTOR ( 'NONE', #9384, 1000.000000000000000 ) ;
#2912=CARTESIAN_POINT ( 'NONE',  ( -5.999999999999999112, 62.00000000000000000, 60.00000000000002132 ) ) ;
#2923=EDGE_LOOP ( 'NONE', ( #12285, #10145 ) ) ;
#2924=DIRECTION ( 'NONE',  ( 0.000000000000000000, 0.000000000000000000, 1.000000000000000000 ) ) ;
#2932=EDGE_CURVE ( 'NONE', #8296, #7815, #1162, .T. ) ;
#2937=DIRECTION ( 'NONE',  ( -0.7236679289129753778, 0.000000000000000000, 0.6901483381584025967 ) ) ;
#2939=EDGE_LOOP ( 'NONE', ( #12230, #8447, #10864, #2891 ) ) ;
#2965=EDGE_CURVE ( 'NONE', #2816, #1278, #6337, .T. ) ;
#2984=EDGE_LOOP ( 'NONE', ( #1803, #9733, #9734, #886 ) ) ;
#2986=ORIENTED_EDGE ( 'NONE', *, *, #3568, .T. ) ;
#2993=VERTEX_POINT ( 'NONE', #5675 ) ;
#2997=ORIENTED_EDGE ( 'NONE', *, *, #1441, .F. ) ;
#3002=VERTEX_POINT ( 'NONE', #109 ) ;
#3005=DIRECTION ( 'NONE',  ( 0.000000000000000000, 1.000000000000000000, 0.000000000000000000 ) ) ;
#3019=ORIENTED_EDGE ( 'NONE', *, *, #3568, .F. ) ;
#3026=CARTESIAN_POINT ( 'NONE',  ( 109.9268209223821628, 275.0000000000000000, 32.26598893414752212 ) ) ;
#3032=DIRECTION ( 'NONE',  ( 0.000000000000000000, 0.000000000000000000, 1.000000000000000000 ) ) ;
#3034=EDGE_CURVE ( 'NONE', #2993, #9781, #9458, .T. ) ;
#3045=EDGE_CURVE ( 'NONE', #1500, #12351, #939, .T. ) ;
#3050=DIRECTION ( 'NONE',  ( -0.9717889794219070065, 0.000000000000000000, -0.2358520287683117111 ) ) ;
#3056=DIRECTION ( 'NONE',  ( 0.000000000000000000, -1.000000000000000000, -0.000000000000000000 ) ) ;
#3063=ORIENTED_EDGE ( 'NONE', *, *, #3034, .F. ) ;
#3066=EDGE_LOOP ( 'NONE', ( #1337, #8361, #7237, #7200 ) ) ;
#3067=LINE ( 'NONE', #11733, #1226 ) ;
#3085=CARTESIAN_POINT ( 'NONE',  ( -89.80805993797480369, 285.0000000000000568, 71.82974571984181011 ) ) ;
#3088=CYLINDRICAL_SURFACE ( 'NONE', #216, 73.00000000000002842 ) ;
#3115=ORIENTED_EDGE ( 'NONE', *, *, #8011, .F. ) ;
#3116=LINE ( 'NONE', #1064, #12055 ) ;
#3150=AXIS2_PLACEMENT_3D ( 'NONE', #3615, #2497, #5555 ) ;
#3152=ORIENTED_EDGE ( 'NONE', *, *, #11598, .T. ) ;
#3153=ORIENTED_EDGE ( 'NONE', *, *, #2932, .F. ) ;
#3171=CARTESIAN_POINT ( 'NONE',  ( 0.000000000000000000, 52.00000000000000711, 0.000000000000000000 ) ) ;
#3174=AXIS2_PLACEMENT_3D ( 'NONE', #127, #2818, #7616 ) ;
#3178=VERTEX_POINT ( 'NONE', #11073 ) ;
#3181=APPLICATION_CONTEXT ( 'automotive_design' ) ;
#3183=CIRCLE ( 'NONE', #4373, 10.00000000000000178 ) ;
#3192=EDGE_LOOP ( 'NONE', ( #8165, #4054, #9076, #504 ) ) ;
#3197=VERTEX_POINT ( 'NONE', #8067 ) ;
#3221=CARTESIAN_POINT ( 'NONE',  ( -82.90657655639077461, 285.0000000000000568, 79.06642500897154946 ) ) ;
#3235=EDGE_LOOP ( 'NONE', ( #11961, #3542, #2491, #1580 ) ) ;
#3253=DIRECTION ( 'NONE',  ( -1.000000000000000000, 0.000000000000000000, 0.000000000000000000 ) ) ;
#3259=CIRCLE ( 'NONE', #10222, 15.00000000000000000 ) ;
#3263=ORIENTED_EDGE ( 'NONE', *, *, #6982, .T. ) ;
#3265=CARTESIAN_POINT ( 'NONE',  ( -89.80805993797480369, 275.0000000000000000, 81.82974571984181011 ) ) ;
#3266=DIRECTION ( 'NONE',  ( 0.000000000000000000, 1.000000000000000000, 0.000000000000000000 ) ) ;
#3269=EDGE_CURVE ( 'NONE', #10685, #7290, #8719, .T. ) ;
#3270=VERTEX_POINT ( 'NONE', #9703 ) ;
#3271=AXIS2_PLACEMENT_3D ( 'NONE', #5451, #6134, #7321 ) ;
#3272=VERTEX_POINT ( 'NONE', #9060 ) ;
#3293=EDGE_CURVE ( 'NONE', #5680, #4162, #594, .T. ) ;
#3295=EDGE_LOOP ( 'NONE', ( #4189, #2130, #5304, #1286, #1935, #6985, #2168 ) ) ;
#3304=AXIS2_PLACEMENT_3D ( 'NONE', #3171, #4053, #7844 ) ;
#3308=EDGE_CURVE ( 'NONE', #2099, #3401, #12317, .T. ) ;
#3311=ORIENTED_EDGE ( 'NONE', *, *, #3420, .T. ) ;
#3314=FACE_OUTER_BOUND ( 'NONE', #2939, .T. ) ;
#3315=ORIENTED_EDGE ( 'NONE', *, *, #11692, .T. ) ;
#3316=SHAPE_REPRESENTATION ( 'Clear Processing Bowl', ( #1612 ), #1360 ) ;
#3323=VECTOR ( 'NONE', #8306, 1000.000000000000000 ) ;
#3328=DIRECTION ( 'NONE',  ( 0.000000000000000000, -0.000000000000000000, 1.000000000000000000 ) ) ;
#3333=CARTESIAN_POINT ( 'NONE',  ( 6.000000000000000000, 62.00000000000000000, 69.74238309665078361 ) ) ;
#3339=( LENGTH_UNIT ( ) NAMED_UNIT ( * ) SI_UNIT ( .MILLI., .METRE. ) );
#3355=CARTESIAN_POINT ( 'NONE',  ( 109.9268209223821628, 275.0000000000000000, 32.26598893414752212 ) ) ;
#3356=AXIS2_PLACEMENT_3D ( 'NONE', #6331, #1473, #5278 ) ;
#3358=ADVANCED_FACE ( 'NONE', ( #12200, #6458 ), #5650, .T. ) ;
#3362=ORIENTED_EDGE ( 'NONE', *, *, #11281, .F. ) ;
#3363=FACE_OUTER_BOUND ( 'NONE', #10278, .T. ) ;
#3364=CARTESIAN_POINT ( 'NONE',  ( -89.80805993797480369, 275.0000000000000000, 71.82974571984181011 ) ) ;
#3400=ORIENTED_EDGE ( 'NONE', *, *, #9873, .T. ) ;
#3401=VERTEX_POINT ( 'NONE', #8496 ) ;
#3402=AXIS2_PLACEMENT_3D ( 'NONE', #1952, #5579, #5703 ) ;
#3409=DIRECTION ( 'NONE',  ( 0.000000000000000000, -1.000000000000000000, -0.000000000000000000 ) ) ;
#3420=EDGE_CURVE ( 'NONE', #6532, #2361, #10111, .T. ) ;
#3425=DIRECTION ( 'NONE',  ( 1.224646799147352961E-16, 0.000000000000000000, -1.000000000000000000 ) ) ;
#3426=DIRECTION ( 'NONE',  ( 0.9595199576812829534, 0.000000000000000000, -0.2816406412634883671 ) ) ;
#3430=AXIS2_PLACEMENT_3D ( 'NONE', #12017, #4462, #11954 ) ;
#3457=EDGE_LOOP ( 'NONE', ( #6158, #8853 ) ) ;
#3459=DIRECTION ( 'NONE',  ( 0.000000000000000000, 1.000000000000000000, 0.000000000000000000 ) ) ;
#3477=DIRECTION ( 'NONE',  ( 0.000000000000000000, 0.000000000000000000, 1.000000000000000000 ) ) ;
#3488=CARTESIAN_POINT ( 'NONE',  ( 0.000000000000000000, 65.00000000000000000, -72.00000000000002842 ) ) ;
#3489=ORIENTED_EDGE ( 'NONE', *, *, #8664, .T. ) ;
#3492=EDGE_LOOP ( 'NONE', ( #851, #7800, #9621, #7866, #3063 ) ) ;
#3493=DIRECTION ( 'NONE',  ( -1.000000000000000000, 0.000000000000000000, 0.000000000000000000 ) ) ;
#3498=FACE_OUTER_BOUND ( 'NONE', #4380, .T. ) ;
#3504=AXIS2_PLACEMENT_3D ( 'NONE', #4659, #10201, #677 ) ;
#3510=AXIS2_PLACEMENT_3D ( 'NONE', #1261, #10034, #4242 ) ;
#3533=FACE_OUTER_BOUND ( 'NONE', #6571, .T. ) ;
#3542=ORIENTED_EDGE ( 'NONE', *, *, #926, .T. ) ;
#3550=LINE ( 'NONE', #9270, #11560 ) ;
#3556=ORIENTED_EDGE ( 'NONE', *, *, #1936, .T. ) ;
#3559=ORIENTED_EDGE ( 'NONE', *, *, #4758, .F. ) ;
#3568=EDGE_CURVE ( 'NONE', #950, #1278, #2207, .T. ) ;
#3574=DIRECTION ( 'NONE',  ( 0.000000000000000000, 1.000000000000000000, 0.000000000000000000 ) ) ;
#3576=DIRECTION ( 'NONE',  ( -0.000000000000000000, -1.000000000000000000, -0.000000000000000000 ) ) ;
#3579=CIRCLE ( 'NONE', #6360, 100.0000000000000142 ) ;
#3580=CIRCLE ( 'NONE', #2581, 90.00000000000002842 ) ;
#3583=EDGE_LOOP ( 'NONE', ( #7601, #7714, #3152, #7925 ) ) ;
#3590=CARTESIAN_POINT ( 'NONE',  ( 109.9268209223821628, 285.0000000000000568, 32.26598893414752212 ) ) ;
#3598=ORIENTED_EDGE ( 'NONE', *, *, #6620, .T. ) ;
#3601=EDGE_CURVE ( 'NONE', #5901, #950, #9655, .T. ) ;
#3605=ORIENTED_EDGE ( 'NONE', *, *, #584, .T. ) ;
#3615=CARTESIAN_POINT ( 'NONE',  ( 0.000000000000000000, 285.0000000000000568, 0.000000000000000000 ) ) ;
#3622=VERTEX_POINT ( 'NONE', #8240 ) ;
#3623=DIRECTION ( 'NONE',  ( 0.000000000000000000, -1.000000000000000000, 0.000000000000000000 ) ) ;
#3626=ORIENTED_EDGE ( 'NONE', *, *, #901, .T. ) ;
#3629=ORIENTED_EDGE ( 'NONE', *, *, #11692, .F. ) ;
#3631=DIRECTION ( 'NONE',  ( 0.000000000000000000, 0.000000000000000000, 1.000000000000000000 ) ) ;
#3637=DIRECTION ( 'NONE',  ( 0.000000000000000000, 0.000000000000000000, -1.000000000000000000 ) ) ;
#3646=VECTOR ( 'NONE', #5294, 1000.000000000000000 ) ;
#3663=DIRECTION ( 'NONE',  ( 0.000000000000000000, -1.000000000000000000, 0.000000000000000000 ) ) ;
#3665=CIRCLE ( 'NONE', #10630, 8.000000000000000000 ) ;
#3675=ORIENTED_EDGE ( 'NONE', *, *, #9455, .F. ) ;
#3683=DIRECTION ( 'NONE',  ( 0.000000000000000000, 1.000000000000000000, 0.000000000000000000 ) ) ;
#3689=ORIENTED_EDGE ( 'NONE', *, *, #9515, .F. ) ;
#3704=CARTESIAN_POINT ( 'NONE',  ( 0.000000000000000000, 265.0000000000000000, 0.000000000000000000 ) ) ;
#3712=DIRECTION ( 'NONE',  ( 0.000000000000000000, 0.000000000000000000, 1.000000000000000000 ) ) ;
#3719=DIRECTION ( 'NONE',  ( 1.000000000000000000, -0.000000000000000000, 1.224646799147353207E-16 ) ) ;
#3720=DIRECTION ( 'NONE',  ( -1.000000000000000000, 0.000000000000000000, 0.000000000000000000 ) ) ;
#3727=DIRECTION ( 'NONE',  ( 0.000000000000000000, 0.000000000000000000, 1.000000000000000000 ) ) ;
#3732=EDGE_LOOP ( 'NONE', ( #145, #8543 ) ) ;
#3742=VECTOR ( 'NONE', #5617, 1000.000000000000000 ) ;
#3744=VERTEX_POINT ( 'NONE', #8669 ) ;
#3752=ORIENTED_EDGE ( 'NONE', *, *, #9309, .F. ) ;
#3765=VECTOR ( 'NONE', #10694, 1000.000000000000000 ) ;
#3773=CARTESIAN_POINT ( 'NONE',  ( 1.285879139104721264E-14, 260.0000000000000000, -105.0000000000000426 ) ) ;
#3775=AXIS2_PLACEMENT_3D ( 'NONE', #8335, #2670, #10396 ) ;
#3781=EDGE_LOOP ( 'NONE', ( #6244, #3855, #10418, #12312 ) ) ;
#3794=DIRECTION ( 'NONE',  ( 0.000000000000000000, 1.000000000000000000, 0.000000000000000000 ) ) ;
#3801=FACE_OUTER_BOUND ( 'NONE', #11494, .T. ) ;
#3803=ORIENTED_EDGE ( 'NONE', *, *, #7194, .F. ) ;
#3807=AXIS2_PLACEMENT_3D ( 'NONE', #4933, #120, #4056 ) ;
#3833=ADVANCED_FACE ( 'NONE', ( #3314 ), #440, .F. ) ;
#3836=AXIS2_PLACEMENT_3D ( 'NONE', #9245, #731, #12012 ) ;
#3838=PLANE ( 'NONE',  #8002 ) ;
#3841=CARTESIAN_POINT ( 'NONE',  ( -5.999999999999999112, 62.00000000000000000, 60.00000000000002132 ) ) ;
#3855=ORIENTED_EDGE ( 'NONE', *, *, #2305, .F. ) ;
#3859=ORIENTED_EDGE ( 'NONE', *, *, #2409, .T. ) ;
#3860=ADVANCED_FACE ( 'NONE', ( #5071 ), #8848, .F. ) ;
#3885=ORIENTED_EDGE ( 'NONE', *, *, #2062, .F. ) ;
#3908=CIRCLE ( 'NONE', #2115, 105.0000000000000426 ) ;
#3919=CARTESIAN_POINT ( 'NONE',  ( 0.000000000000000000, 275.0000000000000000, 0.000000000000000000 ) ) ;
#3920=ADVANCED_FACE ( 'NONE', ( #2314, #6990 ), #4125, .T. ) ;
#3921=CARTESIAN_POINT ( 'NONE',  ( 75.98513253586142469, 275.0000000000000000, 72.46557550663338532 ) ) ;
#3923=DIRECTION ( 'NONE',  ( 0.000000000000000000, 1.000000000000000000, 0.000000000000000000 ) ) ;
#3924=VECTOR ( 'NONE', #10915, 1000.000000000000000 ) ;
#3940=CARTESIAN_POINT ( 'NONE',  ( 0.000000000000000000, 265.0000000000000000, 0.000000000000000000 ) ) ;
#3950=DIRECTION ( 'NONE',  ( -0.000000000000000000, -1.000000000000000000, -0.000000000000000000 ) ) ;
#3961=DIRECTION ( 'NONE',  ( 0.000000000000000000, -0.000000000000000000, 1.000000000000000000 ) ) ;
#3966=ADVANCED_FACE ( 'NONE', ( #3498 ), #4613, .T. ) ;
#3971=FACE_OUTER_BOUND ( 'NONE', #5156, .T. ) ;
#3973=DIRECTION ( 'NONE',  ( 0.000000000000000000, 1.000000000000000000, 0.000000000000000000 ) ) ;
#3975=ORIENTED_EDGE ( 'NONE', *, *, #4758, .T. ) ;
#3976=DIRECTION ( 'NONE',  ( 0.000000000000000000, -0.000000000000000000, 1.000000000000000000 ) ) ;
#3985=AXIS2_PLACEMENT_3D ( 'NONE', #4502, #3253, #11930 ) ;
#3995=ORIENTED_EDGE ( 'NONE', *, *, #9433, .F. ) ;
#4001=DIRECTION ( 'NONE',  ( -0.000000000000000000, -1.000000000000000000, -0.000000000000000000 ) ) ;
#4009=DIRECTION ( 'NONE',  ( 0.000000000000000000, 1.000000000000000000, 0.000000000000000000 ) ) ;
#4014=VECTOR ( 'NONE', #492, 1000.000000000000000 ) ;
#4024=PLANE ( 'NONE',  #2368 ) ;
#4026=AXIS2_PLACEMENT_3D ( 'NONE', #7490, #3683, #11301 ) ;
#4053=DIRECTION ( 'NONE',  ( 0.000000000000000000, 1.000000000000000000, 0.000000000000000000 ) ) ;
#4054=ORIENTED_EDGE ( 'NONE', *, *, #584, .F. ) ;
#4055=LINE ( 'NONE', #1997, #10823 ) ;
#4056=DIRECTION ( 'NONE',  ( 0.9595199576812789566, 0.000000000000000000, 0.2816406412635021894 ) ) ;
#4068=ORIENTED_EDGE ( 'NONE', *, *, #8855, .F. ) ;
#4070=DIRECTION ( 'NONE',  ( 0.000000000000000000, 1.000000000000000000, 0.000000000000000000 ) ) ;
#4071=AXIS2_PLACEMENT_3D ( 'NONE', #6165, #6047, #9015 ) ;
#4076=ADVANCED_FACE ( 'NONE', ( #3801 ), #1894, .F. ) ;
#4078=VERTEX_POINT ( 'NONE', #2802 ) ;
#4082=VERTEX_POINT ( 'NONE', #9586 ) ;
#4083=DIRECTION ( 'NONE',  ( 0.000000000000000000, 0.000000000000000000, 1.000000000000000000 ) ) ;
#4084=FACE_BOUND ( 'NONE', #1405, .T. ) ;
#4094=VECTOR ( 'NONE', #3426, 1000.000000000000114 ) ;
#4100=AXIS2_PLACEMENT_3D ( 'NONE', #1884, #3574, #11250 ) ;
#4101=ORIENTED_EDGE ( 'NONE', *, *, #11893, .T. ) ;
#4104=EDGE_CURVE ( 'NONE', #2993, #2376, #1993, .T. ) ;
#4111=ORIENTED_EDGE ( 'NONE', *, *, #2239, .F. ) ;
#4125=PLANE ( 'NONE',  #9058 ) ;
#4131=CARTESIAN_POINT ( 'NONE',  ( -82.90657655639077461, 275.0000000000000000, 79.06642500897154946 ) ) ;
#4149=( NAMED_UNIT ( * ) SI_UNIT ( $, .STERADIAN. ) SOLID_ANGLE_UNIT ( ) );
#4150=ORIENTED_EDGE ( 'NONE', *, *, #9309, .T. ) ;
#4154=FACE_OUTER_BOUND ( 'NONE', #7451, .T. ) ;
#4162=VERTEX_POINT ( 'NONE', #7785 ) ;
#4164=DIRECTION ( 'NONE',  ( 0.000000000000000000, 1.000000000000000000, 0.000000000000000000 ) ) ;
#4169=CARTESIAN_POINT ( 'NONE',  ( 0.000000000000000000, 65.00000000000000000, 90.00000000000002842 ) ) ;
#4177=DIRECTION ( 'NONE',  ( 0.000000000000000000, 1.000000000000000000, 0.000000000000000000 ) ) ;
#4178=CARTESIAN_POINT ( 'NONE',  ( 3.061616997868383043E-15, 67.00000000000000000, -25.00000000000000000 ) ) ;
#4179=EDGE_CURVE ( 'NONE', #9892, #5904, #87, .T. ) ;
#4181=VECTOR ( 'NONE', #6753, 1000.000000000000000 ) ;
#4189=ORIENTED_EDGE ( 'NONE', *, *, #5828, .T. ) ;
#4193=EDGE_CURVE ( 'NONE', #9087, #3178, #4881, .T. ) ;
#4194=EDGE_LOOP ( 'NONE', ( #6253, #7438 ) ) ;
#4196=CARTESIAN_POINT ( 'NONE',  ( 0.000000000000000000, 65.00000000000000000, 0.000000000000000000 ) ) ;
#4202=ORIENTED_EDGE ( 'NONE', *, *, #10975, .T. ) ;
#4204=CARTESIAN_POINT ( 'NONE',  ( 0.000000000000000000, 75.00000000000001421, 0.000000000000000000 ) ) ;
#4218=CARTESIAN_POINT ( 'NONE',  ( 0.000000000000000000, 265.0000000000000000, 0.000000000000000000 ) ) ;
#4227=ORIENTED_EDGE ( 'NONE', *, *, #10004, .F. ) ;
#4230=CIRCLE ( 'NONE', #1838, 9.999999999999994671 ) ;
#4232=LINE ( 'NONE', #2238, #4014 ) ;
#4237=ORIENTED_EDGE ( 'NONE', *, *, #11667, .F. ) ;
#4240=EDGE_LOOP ( 'NONE', ( #4506, #7187, #4921, #4359 ) ) ;
#4242=DIRECTION ( 'NONE',  ( -0.2358520287683112115, 0.000000000000000000, -0.9717889794219070065 ) ) ;
#4252=ORIENTED_EDGE ( 'NONE', *, *, #8293, .T. ) ;
#4253=PLANE ( 'NONE',  #5673 ) ;
#4254=DIRECTION ( 'NONE',  ( 0.000000000000000000, 0.000000000000000000, 1.000000000000000000 ) ) ;
#4263=DIRECTION ( 'NONE',  ( 0.000000000000000000, 0.000000000000000000, -1.000000000000000000 ) ) ;
#4265=CYLINDRICAL_SURFACE ( 'NONE', #3402, 75.00000000000002842 ) ;
#4270=PRESENTATION_STYLE_ASSIGNMENT (( #1469 ) ) ;
#4279=LINE ( 'NONE', #9694, #2292 ) ;
#4280=PLANE ( 'NONE',  #6102 ) ;
#4282=CARTESIAN_POINT ( 'NONE',  ( -89.80805993797480369, 275.0000000000000000, 81.82974571984181011 ) ) ;
#4286=ORIENTED_EDGE ( 'NONE', *, *, #3308, .T. ) ;
#4292=EDGE_LOOP ( 'NONE', ( #3803, #8683 ) ) ;
#4295=ADVANCED_FACE ( 'NONE', ( #3363 ), #11258, .F. ) ;
#4308=DIRECTION ( 'NONE',  ( -0.000000000000000000, -1.000000000000000000, -0.000000000000000000 ) ) ;
#4312=AXIS2_PLACEMENT_3D ( 'NONE', #2700, #3459, #4514 ) ;
#4315=DIRECTION ( 'NONE',  ( 0.000000000000000000, 1.000000000000000000, 0.000000000000000000 ) ) ;
#4324=ORIENTED_EDGE ( 'NONE', *, *, #12003, .T. ) ;
#4333=DIRECTION ( 'NONE',  ( 0.000000000000000000, 0.000000000000000000, -1.000000000000000000 ) ) ;
#4347=CARTESIAN_POINT ( 'NONE',  ( 89.80805993797383735, 275.0000000000000000, 71.82974571984303225 ) ) ;
#4359=ORIENTED_EDGE ( 'NONE', *, *, #9902, .T. ) ;
#4365=DIRECTION ( 'NONE',  ( 0.000000000000000000, 0.000000000000000000, 1.000000000000000000 ) ) ;
#4373=AXIS2_PLACEMENT_3D ( 'NONE', #8734, #198, #7811 ) ;
#4374=ORIENTED_EDGE ( 'NONE', *, *, #10508, .T. ) ;
#4376=CARTESIAN_POINT ( 'NONE',  ( 0.000000000000000000, 260.0000000000000000, 0.000000000000000000 ) ) ;
#4380=EDGE_LOOP ( 'NONE', ( #233, #4374, #7693, #7848 ) ) ;
#4386=ORIENTED_EDGE ( 'NONE', *, *, #5546, .F. ) ;
#4387=AXIS2_PLACEMENT_3D ( 'NONE', #8810, #6023, #2152 ) ;
#4391=DIRECTION ( 'NONE',  ( -0.000000000000000000, -1.000000000000000000, -0.000000000000000000 ) ) ;
#4395=CARTESIAN_POINT ( 'NONE',  ( -107.1104145097476987, 275.0000000000000000, 41.86118851095882576 ) ) ;
#4433=VERTEX_POINT ( 'NONE', #6415 ) ;
#4445=LINE ( 'NONE', #583, #12271 ) ;
#4446=ADVANCED_FACE ( 'NONE', ( #1674 ), #10839, .T. ) ;
#4454=AXIS2_PLACEMENT_3D ( 'NONE', #11106, #3623, #4676 ) ;
#4462=DIRECTION ( 'NONE',  ( -1.000000000000000000, 0.000000000000000000, -1.224646799147352961E-16 ) ) ;
#4464=ORIENTED_EDGE ( 'NONE', *, *, #9238, .F. ) ;
#4468=EDGE_CURVE ( 'NONE', #11813, #7928, #8391, .T. ) ;
#4470=DIRECTION ( 'NONE',  ( 1.224646799147354193E-16, 0.000000000000000000, -1.000000000000000000 ) ) ;
#4479=EDGE_CURVE ( 'NONE', #5668, #5619, #11090, .T. ) ;
#4482=DIRECTION ( 'NONE',  ( -0.000000000000000000, -1.000000000000000000, -0.000000000000000000 ) ) ;
#4489=AXIS2_PLACEMENT_3D ( 'NONE', #8451, #3973, #4658 ) ;
#4502=CARTESIAN_POINT ( 'NONE',  ( 0.000000000000000000, 75.00000000000001421, 90.00000000000002842 ) ) ;
#4506=ORIENTED_EDGE ( 'NONE', *, *, #4468, .F. ) ;
#4512=ORIENTED_EDGE ( 'NONE', *, *, #4773, .F. ) ;
#4514=DIRECTION ( 'NONE',  ( 0.000000000000000000, 0.000000000000000000, 1.000000000000000000 ) ) ;
#4526=ADVANCED_FACE ( 'NONE', ( #1919 ), #6672, .F. ) ;
#4527=CARTESIAN_POINT ( 'NONE',  ( 6.000000000000000888, 62.00000000000000000, 60.00000000000002132 ) ) ;
#4536=DIRECTION ( 'NONE',  ( 0.000000000000000000, 0.000000000000000000, 1.000000000000000000 ) ) ;
#4539=DIRECTION ( 'NONE',  ( 0.000000000000000000, 0.000000000000000000, 1.000000000000000000 ) ) ;
#4543=ORIENTED_EDGE ( 'NONE', *, *, #11154, .T. ) ;
#4548=EDGE_LOOP ( 'NONE', ( #6796, #9166 ) ) ;
#4551=VERTEX_POINT ( 'NONE', #1851 ) ;
#4563=EDGE_CURVE ( 'NONE', #2554, #9087, #4781, .T. ) ;
#4574=VERTEX_POINT ( 'NONE', #8572 ) ;
#4581=CARTESIAN_POINT ( 'NONE',  ( 0.000000000000000000, 67.00000000000000000, 0.000000000000000000 ) ) ;
#4596=LINE ( 'NONE', #11145, #2456 ) ;
#4613=CYLINDRICAL_SURFACE ( 'NONE', #5511, 75.00000000000002842 ) ;
#4631=ORIENTED_EDGE ( 'NONE', *, *, #5168, .T. ) ;
#4632=LINE ( 'NONE', #6324, #4923 ) ;
#4643=CARTESIAN_POINT ( 'NONE',  ( 116.4243635975512490, 275.0000000000000000, 45.50129185973946022 ) ) ;
#4644=ORIENTED_EDGE ( 'NONE', *, *, #5415, .F. ) ;
#4646=CYLINDRICAL_SURFACE ( 'NONE', #2797, 17.00000000000000000 ) ;
#4652=DIRECTION ( 'NONE',  ( 0.000000000000000000, -1.000000000000000000, 0.000000000000000000 ) ) ;
#4653=DIRECTION ( 'NONE',  ( 0.000000000000000000, 0.000000000000000000, 1.000000000000000000 ) ) ;
#4654=DIRECTION ( 'NONE',  ( 0.000000000000000000, 1.000000000000000000, 0.000000000000000000 ) ) ;
#4657=AXIS2_PLACEMENT_3D ( 'NONE', #6522, #5649, #6576 ) ;
#4658=DIRECTION ( 'NONE',  ( 0.000000000000000000, 0.000000000000000000, 1.000000000000000000 ) ) ;
#4659=CARTESIAN_POINT ( 'NONE',  ( 0.000000000000000000, 50.00000000000000000, 0.000000000000000000 ) ) ;
#4663=ORIENTED_EDGE ( 'NONE', *, *, #9564, .T. ) ;
#4665=AXIS2_PLACEMENT_3D ( 'NONE', #9386, #8454, #10080 ) ;
#4676=DIRECTION ( 'NONE',  ( 0.4999999999999919509, 0.000000000000000000, 0.8660254037844432595 ) ) ;
#4684=ORIENTED_EDGE ( 'NONE', *, *, #8884, .F. ) ;
#4695=VERTEX_POINT ( 'NONE', #5223 ) ;
#4707=CARTESIAN_POINT ( 'NONE',  ( 17.30235457177317571, 285.0000000000000568, -113.6909342308024407 ) ) ;
#4716=PRESENTATION_STYLE_ASSIGNMENT (( #11521 ) ) ;
#4747=AXIS2_PLACEMENT_3D ( 'NONE', #4581, #911, #1658 ) ;
#4758=EDGE_CURVE ( 'NONE', #4939, #8296, #9844, .T. ) ;
#4766=CIRCLE ( 'NONE', #7759, 105.0000000000000426 ) ;
#4767=CIRCLE ( 'NONE', #11743, 9.999999999999994671 ) ;
#4773=EDGE_CURVE ( 'NONE', #3622, #4939, #4279, .T. ) ;
#4775=UNCERTAINTY_MEASURE_WITH_UNIT (LENGTH_MEASURE( 1.000000000000000082E-05 ), #10936, 'distance_accuracy_value', 'NONE');
#4777=( NAMED_UNIT ( * ) PLANE_ANGLE_UNIT ( ) SI_UNIT ( $, .RADIAN. ) );
#4778=ORIENTED_EDGE ( 'NONE', *, *, #2732, .T. ) ;
#4781=LINE ( 'NONE', #5787, #8457 ) ;
#4787=EDGE_LOOP ( 'NONE', ( #10335, #6411, #4663, #10434 ) ) ;
#4788=DIRECTION ( 'NONE',  ( 0.000000000000000000, -1.000000000000000000, 0.000000000000000000 ) ) ;
#4813=EDGE_LOOP ( 'NONE', ( #8218, #4, #2570, #6223 ) ) ;
#4819=VERTEX_POINT ( 'NONE', #2472 ) ;
#4822=DIRECTION ( 'NONE',  ( 0.000000000000000000, 1.000000000000000000, 0.000000000000000000 ) ) ;
#4827=VERTEX_POINT ( 'NONE', #3590 ) ;
#4832=AXIS2_PLACEMENT_3D ( 'NONE', #7575, #9492, #8561 ) ;
#4834=FACE_OUTER_BOUND ( 'NONE', #387, .T. ) ;
#4845=ADVANCED_FACE ( 'NONE', ( #3533 ), #2592, .F. ) ;
#4847=DIRECTION ( 'NONE',  ( 0.000000000000000000, 0.000000000000000000, -1.000000000000000000 ) ) ;
#4859=CARTESIAN_POINT ( 'NONE',  ( 6.000000000000000000, 50.00000000000000000, 70.00000000000001421 ) ) ;
#4868=DIRECTION ( 'NONE',  ( -0.000000000000000000, -1.000000000000000000, -0.000000000000000000 ) ) ;
#4876=ORIENTED_EDGE ( 'NONE', *, *, #7108, .T. ) ;
#4881=CIRCLE ( 'NONE', #493, 105.0000000000000426 ) ;
#4883=AXIS2_PLACEMENT_3D ( 'NONE', #10604, #4001, #10971 ) ;
#4913=SURFACE_SIDE_STYLE ('',( #32 ) ) ;
#4920=DIRECTION ( 'NONE',  ( 0.000000000000000000, 0.000000000000000000, -1.000000000000000000 ) ) ;
#4921=ORIENTED_EDGE ( 'NONE', *, *, #548, .T. ) ;
#4923=VECTOR ( 'NONE', #5391, 1000.000000000000000 ) ;
#4924=ORIENTED_EDGE ( 'NONE', *, *, #11098, .F. ) ;
#4933=CARTESIAN_POINT ( 'NONE',  ( 100.7495955565343451, 275.0000000000000000, 29.57226733266770680 ) ) ;
#4934=ORIENTED_EDGE ( 'NONE', *, *, #7052, .F. ) ;
#4937=ADVANCED_FACE ( 'NONE', ( #5941, #6750 ), #1082, .T. ) ;
#4939=VERTEX_POINT ( 'NONE', #7861 ) ;
#4942=ORIENTED_EDGE ( 'NONE', *, *, #11765, .F. ) ;
#4949=CARTESIAN_POINT ( 'NONE',  ( 0.000000000000000000, 65.00000000000000000, 0.000000000000000000 ) ) ;
#4961=CARTESIAN_POINT ( 'NONE',  ( -109.9268209223825750, 285.0000000000000568, 32.26598893414599445 ) ) ;
#4964=ADVANCED_FACE ( 'NONE', ( #29 ), #413, .T. ) ;
#4969=AXIS2_PLACEMENT_3D ( 'NONE', #5281, #10186, #9061 ) ;
#4970=CARTESIAN_POINT ( 'NONE',  ( 0.000000000000000000, 265.0000000000000000, -98.00000000000001421 ) ) ;
#4979=CARTESIAN_POINT ( 'NONE',  ( 0.000000000000000000, 260.0000000000000000, 105.0000000000000426 ) ) ;
#4985=AXIS2_PLACEMENT_3D ( 'NONE', #1437, #11097, #5303 ) ;
#5003=FACE_OUTER_BOUND ( 'NONE', #2865, .T. ) ;
#5015=AXIS2_PLACEMENT_3D ( 'NONE', #11985, #629, #2501 ) ;
#5017=VECTOR ( 'NONE', #9064, 1000.000000000000000 ) ;
#5031=ORIENTED_EDGE ( 'NONE', *, *, #7494, .F. ) ;
#5032=DIRECTION ( 'NONE',  ( 1.000000000000000000, 0.000000000000000000, 0.000000000000000000 ) ) ;
#5036=EDGE_CURVE ( 'NONE', #7852, #1429, #9912, .T. ) ;
#5044=ORIENTED_EDGE ( 'NONE', *, *, #8703, .F. ) ;
#5049=ORIENTED_EDGE ( 'NONE', *, *, #11667, .T. ) ;
#5051=DIRECTION ( 'NONE',  ( -0.2358520287683116834, 0.000000000000000000, 0.9717889794219068955 ) ) ;
#5056=DIRECTION ( 'NONE',  ( -1.000000000000000000, 0.000000000000000000, 0.000000000000000000 ) ) ;
#5071=FACE_OUTER_BOUND ( 'NONE', #2984, .T. ) ;
#5082=EDGE_LOOP ( 'NONE', ( #5148, #6446, #9398, #10539 ) ) ;
#5088=CARTESIAN_POINT ( 'NONE',  ( 0.000000000000000000, 285.0000000000000568, 0.000000000000000000 ) ) ;
#5096=EDGE_CURVE ( 'NONE', #5565, #12345, #2293, .T. ) ;
#5098=LINE ( 'NONE', #7884, #6894 ) ;
#5101=AXIS2_PLACEMENT_3D ( 'NONE', #2829, #8430, #10366 ) ;
#5110=ADVANCED_FACE ( 'NONE', ( #11042 ), #9850, .F. ) ;
#5115=ORIENTED_EDGE ( 'NONE', *, *, #8199, .T. ) ;
#5117=LINE ( 'NONE', #361, #514 ) ;
#5129=DIRECTION ( 'NONE',  ( 0.000000000000000000, 0.000000000000000000, 1.000000000000000000 ) ) ;
#5131=DIRECTION ( 'NONE',  ( 0.000000000000000000, 0.000000000000000000, 1.000000000000000000 ) ) ;
#5133=EDGE_LOOP ( 'NONE', ( #3885, #6085, #251, #8023 ) ) ;
#5135=EDGE_CURVE ( 'NONE', #4819, #6039, #9248, .T. ) ;
#5142=ORIENTED_EDGE ( 'NONE', *, *, #3601, .F. ) ;
#5148=ORIENTED_EDGE ( 'NONE', *, *, #11274, .F. ) ;
#5156=EDGE_LOOP ( 'NONE', ( #4631, #11808, #6537, #4512 ) ) ;
#5168=EDGE_CURVE ( 'NONE', #3622, #1438, #3259, .T. ) ;
#5170=CARTESIAN_POINT ( 'NONE',  ( 27.02024436599224444, 275.0000000000000000, -111.3324139431193203 ) ) ;
#5175=CIRCLE ( 'NONE', #12148, 98.00000000000001421 ) ;
#5191=DIRECTION ( 'NONE',  ( 0.000000000000000000, 1.000000000000000000, 0.000000000000000000 ) ) ;
#5201=PRODUCT_DEFINITION ( 'UNKNOWN', '', #7344, #1275 ) ;
#5203=DIRECTION ( 'NONE',  ( 0.000000000000000000, 0.000000000000000000, -1.000000000000000000 ) ) ;
#5205=FACE_OUTER_BOUND ( 'NONE', #9502, .T. ) ;
#5207=EDGE_LOOP ( 'NONE', ( #6372, #558 ) ) ;
#5223=CARTESIAN_POINT ( 'NONE',  ( 75.98513253586142469, 285.0000000000000568, 72.46557550663338532 ) ) ;
#5235=EDGE_LOOP ( 'NONE', ( #5921, #7175, #12008, #11404 ) ) ;
#5242=VECTOR ( 'NONE', #9071, 1000.000000000000000 ) ;
#5250=VERTEX_POINT ( 'NONE', #12047 ) ;
#5253=LINE ( 'NONE', #507, #6800 ) ;
#5260=ORIENTED_EDGE ( 'NONE', *, *, #3269, .T. ) ;
#5261=FACE_OUTER_BOUND ( 'NONE', #5207, .T. ) ;
#5263=AXIS2_PLACEMENT_3D ( 'NONE', #11567, #1338, #10803 ) ;
#5276=UNCERTAINTY_MEASURE_WITH_UNIT (LENGTH_MEASURE( 1.000000000000000082E-05 ), #5723, 'distance_accuracy_value', 'NONE');
#5278=DIRECTION ( 'NONE',  ( 0.000000000000000000, 0.000000000000000000, -1.000000000000000000 ) ) ;
#5281=CARTESIAN_POINT ( 'NONE',  ( 0.000000000000000000, 67.00000000000000000, 0.000000000000000000 ) ) ;
#5282=AXIS2_PLACEMENT_3D ( 'NONE', #516, #10862, #9921 ) ;
#5284=CARTESIAN_POINT ( 'NONE',  ( -75.98513253586240523, 275.0000000000000000, 72.46557550663233371 ) ) ;
#5287=ADVANCED_FACE ( 'NONE', ( #8347 ), #12172, .T. ) ;
#5291=DIRECTION ( 'NONE',  ( 0.000000000000000000, 1.000000000000000000, 0.000000000000000000 ) ) ;
#5294=DIRECTION ( 'NONE',  ( 0.000000000000000000, 1.000000000000000000, 0.000000000000000000 ) ) ;
#5298=VERTEX_POINT ( 'NONE', #6552 ) ;
#5300=LINE ( 'NONE', #2489, #12182 ) ;
#5303=DIRECTION ( 'NONE',  ( 0.000000000000000000, 0.000000000000000000, 1.000000000000000000 ) ) ;
#5304=ORIENTED_EDGE ( 'NONE', *, *, #8242, .T. ) ;
#5312=ORIENTED_EDGE ( 'NONE', *, *, #2658, .T. ) ;
#5332=EDGE_CURVE ( 'NONE', #4078, #6640, #4055, .T. ) ;
#5357=DIRECTION ( 'NONE',  ( 0.000000000000000000, 0.000000000000000000, -1.000000000000000000 ) ) ;
#5371=CARTESIAN_POINT ( 'NONE',  ( 0.000000000000000000, 65.00000000000000000, 0.000000000000000000 ) ) ;
#5374=CARTESIAN_POINT ( 'NONE',  ( -24.76446302067273209, 285.0000000000000568, -102.0378428393002679 ) ) ;
#5391=DIRECTION ( 'NONE',  ( 0.000000000000000000, 1.000000000000000000, 0.000000000000000000 ) ) ;
#5405=CARTESIAN_POINT ( 'NONE',  ( 0.000000000000000000, 275.0000000000000000, 0.000000000000000000 ) ) ;
#5408=DIRECTION ( 'NONE',  ( 0.000000000000000000, 0.000000000000000000, 1.000000000000000000 ) ) ;
#5415=EDGE_CURVE ( 'NONE', #5952, #12245, #3116, .T. ) ;
#5417=FACE_OUTER_BOUND ( 'NONE', #6046, .T. ) ;
#5419=DIRECTION ( 'NONE',  ( 0.000000000000000000, 0.000000000000000000, 1.000000000000000000 ) ) ;
#5422=ORIENTED_EDGE ( 'NONE', *, *, #6955, .T. ) ;
#5435=ORIENTED_EDGE ( 'NONE', *, *, #9564, .F. ) ;
#5439=DIRECTION ( 'NONE',  ( -0.000000000000000000, -1.000000000000000000, -0.000000000000000000 ) ) ;
#5446=ADVANCED_FACE ( 'NONE', ( #2867 ), #6673, .T. ) ;
#5451=CARTESIAN_POINT ( 'NONE',  ( 0.000000000000000000, 265.0000000000000000, 0.000000000000000000 ) ) ;
#5456=DIRECTION ( 'NONE',  ( -0.000000000000000000, -1.000000000000000000, -0.000000000000000000 ) ) ;
#5465=CARTESIAN_POINT ( 'NONE',  ( 3.061616997868383043E-15, 75.00000000000001421, -25.00000000000000000 ) ) ;
#5474=CARTESIAN_POINT ( 'NONE',  ( 2.081899558550500280E-15, 75.00000000000001421, 17.00000000000000000 ) ) ;
#5484=DIRECTION ( 'NONE',  ( -0.000000000000000000, -1.000000000000000000, -0.000000000000000000 ) ) ;
#5491=EDGE_LOOP ( 'NONE', ( #8910, #3263, #5940, #4286 ) ) ;
#5497=DIRECTION ( 'NONE',  ( -0.000000000000000000, -1.000000000000000000, -0.000000000000000000 ) ) ;
#5503=CARTESIAN_POINT ( 'NONE',  ( 17.30235457177317571, 275.0000000000000000, -113.6909342308024407 ) ) ;
#5511=AXIS2_PLACEMENT_3D ( 'NONE', #5371, #12290, #11104 ) ;
#5524=AXIS2_PLACEMENT_3D ( 'NONE', #8364, #9171, #2639 ) ;
#5531=PLANE ( 'NONE',  #12162 ) ;
#5537=CARTESIAN_POINT ( 'NONE',  ( 1.163414459189985801E-14, 65.00000000000000000, -90.00000000000002842 ) ) ;
#5538=CARTESIAN_POINT ( 'NONE',  ( 1.102182119232618227E-14, 75.00000000000001421, -90.00000000000002842 ) ) ;
#5546=EDGE_CURVE ( 'NONE', #12245, #2361, #3665, .T. ) ;
#5548=EDGE_CURVE ( 'NONE', #6039, #8739, #474, .T. ) ;
#5555=DIRECTION ( 'NONE',  ( 0.000000000000000000, 0.000000000000000000, 1.000000000000000000 ) ) ;
#5562=DIRECTION ( 'NONE',  ( 0.000000000000000000, 1.000000000000000000, 0.000000000000000000 ) ) ;
#5564=CARTESIAN_POINT ( 'NONE',  ( -27.02024436599226576, 275.0000000000000000, -111.3324139431193345 ) ) ;
#5565=VERTEX_POINT ( 'NONE', #4169 ) ;
#5579=DIRECTION ( 'NONE',  ( -0.000000000000000000, -1.000000000000000000, -0.000000000000000000 ) ) ;
#5605=CARTESIAN_POINT ( 'NONE',  ( 8.817456953860944867E-15, 65.00000000000000000, 72.00000000000002842 ) ) ;
#5609=CYLINDRICAL_SURFACE ( 'NONE', #5664, 72.00000000000002842 ) ;
#5610=CARTESIAN_POINT ( 'NONE',  ( 0.000000000000000000, 285.0000000000000568, 0.000000000000000000 ) ) ;
#5612=VERTEX_POINT ( 'NONE', #7475 ) ;
#5616=TOROIDAL_SURFACE ( 'NONE', #7407, 25.00000000000000000, 8.000000000000000000 ) ;
#5617=DIRECTION ( 'NONE',  ( -0.000000000000000000, -1.000000000000000000, -0.000000000000000000 ) ) ;
#5619=VERTEX_POINT ( 'NONE', #2667 ) ;
#5630=AXIS2_PLACEMENT_3D ( 'NONE', #2577, #1526, #11061 ) ;
#5644=VERTEX_POINT ( 'NONE', #8395 ) ;
#5645=ORIENTED_EDGE ( 'NONE', *, *, #6982, .F. ) ;
#5649=DIRECTION ( 'NONE',  ( 0.000000000000000000, -1.000000000000000000, -0.000000000000000000 ) ) ;
#5650=PLANE ( 'NONE',  #2160 ) ;
#5663=AXIS2_PLACEMENT_3D ( 'NONE', #11691, #7817, #1093 ) ;
#5664=AXIS2_PLACEMENT_3D ( 'NONE', #679, #12217, #7292 ) ;
#5668=VERTEX_POINT ( 'NONE', #8332 ) ;
#5673=AXIS2_PLACEMENT_3D ( 'NONE', #4196, #8982, #9799 ) ;
#5675=CARTESIAN_POINT ( 'NONE',  ( 6.000000000000000000, 50.00000000000000000, 69.74238309665078361 ) ) ;
#5680=VERTEX_POINT ( 'NONE', #6478 ) ;
#5698=CIRCLE ( 'NONE', #107, 75.00000000000002842 ) ;
#5703=DIRECTION ( 'NONE',  ( 0.000000000000000000, 0.000000000000000000, -1.000000000000000000 ) ) ;
#5704=ADVANCED_FACE ( 'NONE', ( #10267 ), #5609, .T. ) ;
#5710=VERTEX_POINT ( 'NONE', #11285 ) ;
#5716=AXIS2_PLACEMENT_3D ( 'NONE', #1343, #3266, #6201 ) ;
#5723=( LENGTH_UNIT ( ) NAMED_UNIT ( * ) SI_UNIT ( .MILLI., .METRE. ) );
#5725=EDGE_CURVE ( 'NONE', #5612, #6532, #8237, .T. ) ;
#5734=CARTESIAN_POINT ( 'NONE',  ( 0.000000000000000000, 65.00000000000000000, 0.000000000000000000 ) ) ;
#5738=ORIENTED_EDGE ( 'NONE', *, *, #6955, .F. ) ;
#5744=DIRECTION ( 'NONE',  ( -1.000000000000000000, 0.000000000000000000, -0.000000000000000000 ) ) ;
#5779=CARTESIAN_POINT ( 'NONE',  ( 0.000000000000000000, 75.00000000000001421, -98.00000000000001421 ) ) ;
#5785=CARTESIAN_POINT ( 'NONE',  ( -24.76446302067273209, 275.0000000000000000, -102.0378428393002679 ) ) ;
#5787=CARTESIAN_POINT ( 'NONE',  ( 100.7495955565343451, 275.0000000000000000, 29.57226733266770680 ) ) ;
#5790=PLANE ( 'NONE',  #894 ) ;
#5802=DIRECTION ( 'NONE',  ( 0.000000000000000000, 0.000000000000000000, 1.000000000000000000 ) ) ;
#5807=CARTESIAN_POINT ( 'NONE',  ( 0.000000000000000000, 75.00000000000001421, -100.0000000000000142 ) ) ;
#5811=AXIS2_PLACEMENT_3D ( 'NONE', #5405, #10249, #7458 ) ;
#5821=ADVANCED_FACE ( 'NONE', ( #231, #38 ), #5790, .T. ) ;
#5828=EDGE_CURVE ( 'NONE', #9195, #5986, #7850, .T. ) ;
#5834=AXIS2_PLACEMENT_3D ( 'NONE', #1034, #8624, #8498 ) ;
#5835=ORIENTED_EDGE ( 'NONE', *, *, #2156, .F. ) ;
#5853=EDGE_LOOP ( 'NONE', ( #12325, #5422, #7172, #6266 ) ) ;
#5860=EDGE_LOOP ( 'NONE', ( #6852, #4924, #5049, #10282 ) ) ;
#5863=ORIENTED_EDGE ( 'NONE', *, *, #8017, .T. ) ;
#5880=CARTESIAN_POINT ( 'NONE',  ( 89.80805993797383735, 275.0000000000000000, 71.82974571984303225 ) ) ;
#5892=ORIENTED_EDGE ( 'NONE', *, *, #2688, .F. ) ;
#5896=CYLINDRICAL_SURFACE ( 'NONE', #5834, 15.00000000000000000 ) ;
#5901=VERTEX_POINT ( 'NONE', #166 ) ;
#5904=VERTEX_POINT ( 'NONE', #2789 ) ;
#5920=LINE ( 'NONE', #9704, #1055 ) ;
#5921=ORIENTED_EDGE ( 'NONE', *, *, #1456, .F. ) ;
#5940=ORIENTED_EDGE ( 'NONE', *, *, #6484, .F. ) ;
#5941=FACE_BOUND ( 'NONE', #10861, .T. ) ;
#5949=EDGE_CURVE ( 'NONE', #2323, #2602, #6218, .T. ) ;
#5952=VERTEX_POINT ( 'NONE', #5969 ) ;
#5959=FACE_OUTER_BOUND ( 'NONE', #8517, .T. ) ;
#5965=DIRECTION ( 'NONE',  ( -0.2358520287683112115, 0.000000000000000000, -0.9717889794219070065 ) ) ;
#5969=CARTESIAN_POINT ( 'NONE',  ( 2.081899558550500280E-15, 115.0000000000000142, 17.00000000000000000 ) ) ;
#5975=DIRECTION ( 'NONE',  ( -0.000000000000000000, -1.000000000000000000, -0.000000000000000000 ) ) ;
#5976=STYLED_ITEM ( 'NONE', ( #4716 ), #461 ) ;
#5986=VERTEX_POINT ( 'NONE', #2287 ) ;
#5992=AXIS2_PLACEMENT_3D ( 'NONE', #5734, #5975, #11471 ) ;
#5995=CARTESIAN_POINT ( 'NONE',  ( -89.80805993797480369, 285.0000000000000568, 71.82974571984181011 ) ) ;
#5998=CARTESIAN_POINT ( 'NONE',  ( -100.7495955565347572, 285.0000000000000568, 29.57226733266631769 ) ) ;
#6001=ORIENTED_EDGE ( 'NONE', *, *, #11148, .T. ) ;
#6016=CARTESIAN_POINT ( 'NONE',  ( 0.000000000000000000, 260.0000000000000000, 100.0000000000000284 ) ) ;
#6022=CARTESIAN_POINT ( 'NONE',  ( 29.48150359603894088, 285.0000000000000568, -121.4736224277384053 ) ) ;
#6023=DIRECTION ( 'NONE',  ( 0.000000000000000000, 1.000000000000000000, 0.000000000000000000 ) ) ;
#6031=CARTESIAN_POINT ( 'NONE',  ( 107.1104145097471445, 275.0000000000000000, 41.86118851096031079 ) ) ;
#6039=VERTEX_POINT ( 'NONE', #666 ) ;
#6040=VECTOR ( 'NONE', #11213, 1000.000000000000000 ) ;
#6044=DIRECTION ( 'NONE',  ( 0.000000000000000000, 0.000000000000000000, 1.000000000000000000 ) ) ;
#6046=EDGE_LOOP ( 'NONE', ( #3675, #3115, #11546, #5738 ) ) ;
#6047=DIRECTION ( 'NONE',  ( 1.000000000000000000, -0.000000000000000000, 1.224646799147353207E-16 ) ) ;
#6049=ORIENTED_EDGE ( 'NONE', *, *, #9054, .T. ) ;
#6057=EDGE_LOOP ( 'NONE', ( #9585, #3859, #4324, #4252, #906 ) ) ;
#6060=VERTEX_POINT ( 'NONE', #8134 ) ;
#6064=ORIENTED_EDGE ( 'NONE', *, *, #7316, .F. ) ;
#6080=ADVANCED_FACE ( 'NONE', ( #7926 ), #1271, .T. ) ;
#6082=AXIS2_PLACEMENT_3D ( 'NONE', #6906, #8999, #1232 ) ;
#6084=ORIENTED_EDGE ( 'NONE', *, *, #10004, .T. ) ;
#6085=ORIENTED_EDGE ( 'NONE', *, *, #154, .F. ) ;
#6102=AXIS2_PLACEMENT_3D ( 'NONE', #5284, #8883, #2286 ) ;
#6103=ADVANCED_FACE ( 'NONE', ( #5261, #1335 ), #4253, .F. ) ;
#6107=ORIENTED_EDGE ( 'NONE', *, *, #5548, .T. ) ;
#6118=ORIENTED_EDGE ( 'NONE', *, *, #8600, .T. ) ;
#6120=CARTESIAN_POINT ( 'NONE',  ( 0.000000000000000000, 67.00000000000000000, 0.000000000000000000 ) ) ;
#6134=DIRECTION ( 'NONE',  ( -0.000000000000000000, -1.000000000000000000, -0.000000000000000000 ) ) ;
#6142=( GEOMETRIC_REPRESENTATION_CONTEXT ( 3 ) GLOBAL_UNCERTAINTY_ASSIGNED_CONTEXT ( ( #4775 ) ) GLOBAL_UNIT_ASSIGNED_CONTEXT ( ( #10936, #9056, #7199 ) ) REPRESENTATION_CONTEXT ( 'NONE', 'WORKASPACE' ) );
#6155=LINE ( 'NONE', #9068, #8164 ) ;
#6158=ORIENTED_EDGE ( 'NONE', *, *, #4179, .T. ) ;
#6159=CARTESIAN_POINT ( 'NONE',  ( 97.61745645431939522, 275.0000000000000000, 78.07581056504676553 ) ) ;
#6165=CARTESIAN_POINT ( 'NONE',  ( 1.102182119232618227E-14, 75.00000000000001421, -90.00000000000002842 ) ) ;
#6168=EDGE_CURVE ( 'NONE', #12189, #6826, #9837, .T. ) ;
#6171=CARTESIAN_POINT ( 'NONE',  ( 0.000000000000000000, 265.0000000000000000, -100.0000000000000142 ) ) ;
#6177=ORIENTED_EDGE ( 'NONE', *, *, #7726, .T. ) ;
#6179=DIRECTION ( 'NONE',  ( 0.000000000000000000, -0.000000000000000000, 1.000000000000000000 ) ) ;
#6180=EDGE_LOOP ( 'NONE', ( #3362, #6427, #3598, #4237 ) ) ;
#6182=DIRECTION ( 'NONE',  ( -0.5000000000000012212, 0.000000000000000000, -0.8660254037844379305 ) ) ;
#6189=CIRCLE ( 'NONE', #7, 125.0000000000000568 ) ;
#6193=ORIENTED_EDGE ( 'NONE', *, *, #6398, .T. ) ;
#6195=DIRECTION ( 'NONE',  ( 0.000000000000000000, 1.000000000000000000, 0.000000000000000000 ) ) ;
#6196=EDGE_CURVE ( 'NONE', #5619, #8739, #285, .T. ) ;
#6201=DIRECTION ( 'NONE',  ( 0.000000000000000000, 0.000000000000000000, 1.000000000000000000 ) ) ;
#6207=SHAPE_REPRESENTATION_RELATIONSHIP ( 'NONE' , 'NONE' ,  #3316, #8978 ) ;
#6218=LINE ( 'NONE', #4282, #8829 ) ;
#6223=ORIENTED_EDGE ( 'NONE', *, *, #6888, .F. ) ;
#6228=ORIENTED_EDGE ( 'NONE', *, *, #2875, .T. ) ;
#6230=ADVANCED_FACE ( 'NONE', ( #2382 ), #2452, .F. ) ;
#6242=CARTESIAN_POINT ( 'NONE',  ( 1.224646799147353375E-14, 75.00000000000001421, 100.0000000000000142 ) ) ;
#6244=ORIENTED_EDGE ( 'NONE', *, *, #435, .F. ) ;
#6253=ORIENTED_EDGE ( 'NONE', *, *, #7802, .F. ) ;
#6266=ORIENTED_EDGE ( 'NONE', *, *, #8397, .F. ) ;
#6273=CARTESIAN_POINT ( 'NONE',  ( 0.000000000000000000, 260.0000000000000000, -100.0000000000000142 ) ) ;
#6291=ORIENTED_EDGE ( 'NONE', *, *, #11796, .F. ) ;
#6303=VECTOR ( 'NONE', #6764, 1000.000000000000000 ) ;
#6312=DIRECTION ( 'NONE',  ( 0.000000000000000000, 1.000000000000000000, 0.000000000000000000 ) ) ;
#6314=VECTOR ( 'NONE', #7744, 1000.000000000000000 ) ;
#6324=CARTESIAN_POINT ( 'NONE',  ( -97.61745645432043261, 275.0000000000000000, 78.07581056504542971 ) ) ;
#6331=CARTESIAN_POINT ( 'NONE',  ( 0.000000000000000000, 275.0000000000000000, 0.000000000000000000 ) ) ;
#6337=CIRCLE ( 'NONE', #152, 100.0000000000000284 ) ;
#6338=CARTESIAN_POINT ( 'NONE',  ( 1.836970198721029589E-15, 265.0000000000000000, 15.00000000000000000 ) ) ;
#6346=CARTESIAN_POINT ( 'NONE',  ( 0.000000000000000000, 265.0000000000000000, 0.000000000000000000 ) ) ;
#6355=EDGE_LOOP ( 'NONE', ( #7120, #11247, #417, #2096 ) ) ;
#6360=AXIS2_PLACEMENT_3D ( 'NONE', #11287, #8333, #4539 ) ;
#6363=CIRCLE ( 'NONE', #992, 10.00000000000000178 ) ;
#6365=CARTESIAN_POINT ( 'NONE',  ( 0.000000000000000000, 65.00000000000000000, -75.00000000000002842 ) ) ;
#6372=ORIENTED_EDGE ( 'NONE', *, *, #5096, .T. ) ;
#6374=DIRECTION ( 'NONE',  ( -0.000000000000000000, -1.000000000000000000, -0.000000000000000000 ) ) ;
#6382=CARTESIAN_POINT ( 'NONE',  ( 0.000000000000000000, 75.00000000000001421, 0.000000000000000000 ) ) ;
#6392=FACE_OUTER_BOUND ( 'NONE', #6668, .T. ) ;
#6397=DIRECTION ( 'NONE',  ( 0.000000000000000000, -1.000000000000000000, -0.000000000000000000 ) ) ;
#6398=EDGE_CURVE ( 'NONE', #4078, #3197, #8643, .T. ) ;
#6404=ORIENTED_EDGE ( 'NONE', *, *, #9179, .T. ) ;
#6409=AXIS2_PLACEMENT_3D ( 'NONE', #7702, #86, #3712 ) ;
#6411=ORIENTED_EDGE ( 'NONE', *, *, #770, .T. ) ;
#6415=CARTESIAN_POINT ( 'NONE',  ( -24.76446302067273564, 285.0000000000000568, -102.0378428393002679 ) ) ;
#6425=DIRECTION ( 'NONE',  ( 0.000000000000000000, 1.000000000000000000, 0.000000000000000000 ) ) ;
#6427=ORIENTED_EDGE ( 'NONE', *, *, #10951, .T. ) ;
#6446=ORIENTED_EDGE ( 'NONE', *, *, #12178, .T. ) ;
#6458=FACE_OUTER_BOUND ( 'NONE', #10995, .T. ) ;
#6473=CARTESIAN_POINT ( 'NONE',  ( 0.000000000000000000, 65.00000000000000000, -73.00000000000002842 ) ) ;
#6476=DIRECTION ( 'NONE',  ( 0.000000000000000000, 0.000000000000000000, -1.000000000000000000 ) ) ;
#6478=CARTESIAN_POINT ( 'NONE',  ( 27.02024436599224444, 275.0000000000000000, -111.3324139431193203 ) ) ;
#6482=CARTESIAN_POINT ( 'NONE',  ( -6.000000000000000000, 50.00000000000000000, 69.74238309665079782 ) ) ;
#6483=AXIS2_PLACEMENT_3D ( 'NONE', #7055, #11926, #505 ) ;
#6484=EDGE_CURVE ( 'NONE', #2099, #2436, #10842, .T. ) ;
#6490=ORIENTED_EDGE ( 'NONE', *, *, #1441, .T. ) ;
#6501=EDGE_LOOP ( 'NONE', ( #5142, #8644, #8020, #3019 ) ) ;
#6516=AXIS2_PLACEMENT_3D ( 'NONE', #1023, #4822, #7562 ) ;
#6517=FACE_OUTER_BOUND ( 'NONE', #1628, .T. ) ;
#6522=CARTESIAN_POINT ( 'NONE',  ( -89.80805993797480369, 275.0000000000000000, 71.82974571984181011 ) ) ;
#6523=DIRECTION ( 'NONE',  ( -0.2358520287683116834, 0.000000000000000000, 0.9717889794219068955 ) ) ;
#6525=DIRECTION ( 'NONE',  ( 0.000000000000000000, 0.000000000000000000, 1.000000000000000000 ) ) ;
#6526=CARTESIAN_POINT ( 'NONE',  ( 8.817456953860944867E-15, 52.00000000000000711, 72.00000000000002842 ) ) ;
#6532=VERTEX_POINT ( 'NONE', #4178 ) ;
#6537=ORIENTED_EDGE ( 'NONE', *, *, #154, .T. ) ;
#6552=CARTESIAN_POINT ( 'NONE',  ( 97.61745645431939522, 285.0000000000000568, 78.07581056504676553 ) ) ;
#6566=DIRECTION ( 'NONE',  ( 0.000000000000000000, 0.000000000000000000, -1.000000000000000000 ) ) ;
#6571=EDGE_LOOP ( 'NONE', ( #2515, #6646, #10925, #1490 ) ) ;
#6576=DIRECTION ( 'NONE',  ( 0.000000000000000000, 0.000000000000000000, -1.000000000000000000 ) ) ;
#6580=DIRECTION ( 'NONE',  ( 0.000000000000000000, 0.000000000000000000, 1.000000000000000000 ) ) ;
#6592=DIRECTION ( 'NONE',  ( -0.000000000000000000, -1.000000000000000000, -0.000000000000000000 ) ) ;
#6594=CARTESIAN_POINT ( 'NONE',  ( 24.76446302067270722, 275.0000000000000000, -102.0378428393002679 ) ) ;
#6601=VECTOR ( 'NONE', #2937, 1000.000000000000000 ) ;
#6613=LINE ( 'NONE', #9590, #6601 ) ;
#6620=EDGE_CURVE ( 'NONE', #1577, #10879, #1254, .T. ) ;
#6621=DIRECTION ( 'NONE',  ( 0.000000000000000000, 0.000000000000000000, 1.000000000000000000 ) ) ;
#6640=VERTEX_POINT ( 'NONE', #11410 ) ;
#6642=DIRECTION ( 'NONE',  ( 1.224646799147352714E-16, 0.000000000000000000, -1.000000000000000000 ) ) ;
#6646=ORIENTED_EDGE ( 'NONE', *, *, #8965, .T. ) ;
#6666=DIRECTION ( 'NONE',  ( 1.224646799147352961E-16, 0.000000000000000000, -1.000000000000000000 ) ) ;
#6668=EDGE_LOOP ( 'NONE', ( #3629, #4876, #6177, #11936 ) ) ;
#6669=DIRECTION ( 'NONE',  ( 0.000000000000000000, 1.000000000000000000, 0.000000000000000000 ) ) ;
#6672=TOROIDAL_SURFACE ( 'NONE', #4489, 90.00000000000002842, 8.000000000000000000 ) ;
#6673=PLANE ( 'NONE',  #11459 ) ;
#6688=AXIS2_PLACEMENT_3D ( 'NONE', #8180, #12350, #9521 ) ;
#6692=LINE ( 'NONE', #1083, #6314 ) ;
#6699=EDGE_LOOP ( 'NONE', ( #9477, #11821, #2677, #1944, #8464, #4202, #7418 ) ) ;
#6704=ORIENTED_EDGE ( 'NONE', *, *, #11318, .T. ) ;
#6721=CARTESIAN_POINT ( 'NONE',  ( 0.000000000000000000, 260.0000000000000000, 0.000000000000000000 ) ) ;
#6729=ORIENTED_EDGE ( 'NONE', *, *, #10963, .F. ) ;
#6732=ORIENTED_EDGE ( 'NONE', *, *, #7726, .F. ) ;
#6739=ORIENTED_EDGE ( 'NONE', *, *, #9902, .F. ) ;
#6742=ORIENTED_EDGE ( 'NONE', *, *, #8751, .T. ) ;
#6750=FACE_OUTER_BOUND ( 'NONE', #2923, .T. ) ;
#6752=DIRECTION ( 'NONE',  ( 0.000000000000000000, 0.000000000000000000, 1.000000000000000000 ) ) ;
#6753=DIRECTION ( 'NONE',  ( -0.000000000000000000, -1.000000000000000000, -0.000000000000000000 ) ) ;
#6759=ORIENTED_EDGE ( 'NONE', *, *, #8017, .F. ) ;
#6763=LINE ( 'NONE', #147, #1780 ) ;
#6764=DIRECTION ( 'NONE',  ( 0.000000000000000000, 1.000000000000000000, 0.000000000000000000 ) ) ;
#6782=DIRECTION ( 'NONE',  ( 0.000000000000000000, 1.000000000000000000, 0.000000000000000000 ) ) ;
#6783=ORIENTED_EDGE ( 'NONE', *, *, #2875, .F. ) ;
#6788=EDGE_CURVE ( 'NONE', #10214, #4082, #2448, .T. ) ;
#6795=FACE_OUTER_BOUND ( 'NONE', #9652, .T. ) ;
#6796=ORIENTED_EDGE ( 'NONE', *, *, #7250, .T. ) ;
#6797=AXIS2_PLACEMENT_3D ( 'NONE', #10215, #5497, #4847 ) ;
#6800=VECTOR ( 'NONE', #4308, 1000.000000000000000 ) ;
#6801=CARTESIAN_POINT ( 'NONE',  ( 0.000000000000000000, 65.00000000000000000, 0.000000000000000000 ) ) ;
#6811=FACE_OUTER_BOUND ( 'NONE', #5082, .T. ) ;
#6826=VERTEX_POINT ( 'NONE', #2054 ) ;
#6829=CARTESIAN_POINT ( 'NONE',  ( -6.000000000000000000, 62.00000000000000000, 69.74238309665079782 ) ) ;
#6849=ADVANCED_FACE ( 'NONE', ( #10468 ), #6915, .F. ) ;
#6852=ORIENTED_EDGE ( 'NONE', *, *, #10951, .F. ) ;
#6861=FACE_OUTER_BOUND ( 'NONE', #11396, .T. ) ;
#6864=ORIENTED_EDGE ( 'NONE', *, *, #2239, .T. ) ;
#6877=CARTESIAN_POINT ( 'NONE',  ( -97.61745645432043261, 275.0000000000000000, 78.07581056504542971 ) ) ;
#6888=EDGE_CURVE ( 'NONE', #108, #1518, #5920, .T. ) ;
#6891=DIRECTION ( 'NONE',  ( 0.000000000000000000, 1.000000000000000000, 0.000000000000000000 ) ) ;
#6894=VECTOR ( 'NONE', #9935, 1000.000000000000000 ) ;
#6898=AXIS2_PLACEMENT_3D ( 'NONE', #3364, #4164, #617 ) ;
#6903=CARTESIAN_POINT ( 'NONE',  ( 1.285879139104721264E-14, 275.0000000000000000, -105.0000000000000426 ) ) ;
#6906=CARTESIAN_POINT ( 'NONE',  ( 0.000000000000000000, 75.00000000000001421, 0.000000000000000000 ) ) ;
#6915=PLANE ( 'NONE',  #456 ) ;
#6935=EDGE_LOOP ( 'NONE', ( #3559, #9625, #10422, #3153 ) ) ;
#6955=EDGE_CURVE ( 'NONE', #5680, #693, #8019, .T. ) ;
#6962=DIRECTION ( 'NONE',  ( -0.000000000000000000, -1.000000000000000000, -0.000000000000000000 ) ) ;
#6965=CIRCLE ( 'NONE', #4985, 72.00000000000002842 ) ;
#6982=EDGE_CURVE ( 'NONE', #5298, #2436, #10895, .T. ) ;
#6985=ORIENTED_EDGE ( 'NONE', *, *, #761, .T. ) ;
#6990=FACE_OUTER_BOUND ( 'NONE', #10466, .T. ) ;
#7006=ADVANCED_FACE ( 'NONE', ( #9010 ), #8082, .T. ) ;
#7012=DIRECTION ( 'NONE',  ( 0.000000000000000000, -0.000000000000000000, 1.000000000000000000 ) ) ;
#7013=LINE ( 'NONE', #6022, #1332 ) ;
#7014=CARTESIAN_POINT ( 'NONE',  ( 0.000000000000000000, 65.00000000000000000, 0.000000000000000000 ) ) ;
#7021=DIRECTION ( 'NONE',  ( 0.000000000000000000, 0.000000000000000000, 1.000000000000000000 ) ) ;
#7034=EDGE_CURVE ( 'NONE', #2259, #1429, #2604, .T. ) ;
#7039=CARTESIAN_POINT ( 'NONE',  ( 100.7495955565343451, 275.0000000000000000, 29.57226733266770680 ) ) ;
#7040=EDGE_CURVE ( 'NONE', #11519, #9781, #4596, .T. ) ;
#7044=AXIS2_PLACEMENT_3D ( 'NONE', #9153, #633, #11736 ) ;
#7049=EDGE_LOOP ( 'NONE', ( #9301, #7294, #6704, #5835, #12349, #3556, #12113, #8862, #4942, #5260 ) ) ;
#7052=EDGE_CURVE ( 'NONE', #3002, #9892, #2661, .T. ) ;
#7055=CARTESIAN_POINT ( 'NONE',  ( 0.000000000000000000, 65.00000000000000000, 0.000000000000000000 ) ) ;
#7073=FACE_OUTER_BOUND ( 'NONE', #7049, .T. ) ;
#7078=ORIENTED_EDGE ( 'NONE', *, *, #8297, .F. ) ;
#7079=FILL_AREA_STYLE_COLOUR ( '', #10132 ) ;
#7094=VERTEX_POINT ( 'NONE', #8389 ) ;
#7108=EDGE_CURVE ( 'NONE', #3272, #2243, #803, .T. ) ;
#7109=ORIENTED_EDGE ( 'NONE', *, *, #8664, .F. ) ;
#7115=CARTESIAN_POINT ( 'NONE',  ( 6.000000000000000000, 62.00000000000000000, 70.00000000000001421 ) ) ;
#7120=ORIENTED_EDGE ( 'NONE', *, *, #2494, .F. ) ;
#7132=DIRECTION ( 'NONE',  ( 0.000000000000000000, 1.000000000000000000, 0.000000000000000000 ) ) ;
#7133=CYLINDRICAL_SURFACE ( 'NONE', #2714, 105.0000000000000426 ) ;
#7166=EDGE_CURVE ( 'NONE', #950, #5901, #1266, .T. ) ;
#7172=ORIENTED_EDGE ( 'NONE', *, *, #8884, .T. ) ;
#7175=ORIENTED_EDGE ( 'NONE', *, *, #5949, .T. ) ;
#7187=ORIENTED_EDGE ( 'NONE', *, *, #8703, .T. ) ;
#7190=DIRECTION ( 'NONE',  ( 0.000000000000000000, 1.000000000000000000, 0.000000000000000000 ) ) ;
#7192=VERTEX_POINT ( 'NONE', #2912 ) ;
#7194=EDGE_CURVE ( 'NONE', #12351, #10877, #262, .T. ) ;
#7199=( NAMED_UNIT ( * ) SI_UNIT ( $, .STERADIAN. ) SOLID_ANGLE_UNIT ( ) );
#7200=ORIENTED_EDGE ( 'NONE', *, *, #7194, .T. ) ;
#7201=AXIS2_PLACEMENT_3D ( 'NONE', #4395, #6397, #8191 ) ;
#7204=CIRCLE ( 'NONE', #631, 9.999999999999994671 ) ;
#7221=ORIENTED_EDGE ( 'NONE', *, *, #6168, .F. ) ;
#7228=EDGE_CURVE ( 'NONE', #10685, #6060, #7710, .T. ) ;
#7237=ORIENTED_EDGE ( 'NONE', *, *, #3045, .T. ) ;
#7238=DIRECTION ( 'NONE',  ( 0.000000000000000000, 0.000000000000000000, 1.000000000000000000 ) ) ;
#7240=ORIENTED_EDGE ( 'NONE', *, *, #5828, .F. ) ;
#7250=EDGE_CURVE ( 'NONE', #1500, #5250, #874, .T. ) ;
#7254=CIRCLE ( 'NONE', #4657, 10.00000000000000178 ) ;
#7260=DIRECTION ( 'NONE',  ( -0.000000000000000000, -1.000000000000000000, -0.000000000000000000 ) ) ;
#7261=CARTESIAN_POINT ( 'NONE',  ( 0.000000000000000000, 265.0000000000000000, 0.000000000000000000 ) ) ;
#7272=VECTOR ( 'NONE', #2485, 1000.000000000000000 ) ;
#7274=VECTOR ( 'NONE', #5191, 1000.000000000000000 ) ;
#7288=DIRECTION ( 'NONE',  ( 0.000000000000000000, 1.000000000000000000, 0.000000000000000000 ) ) ;
#7290=VERTEX_POINT ( 'NONE', #6903 ) ;
#7292=DIRECTION ( 'NONE',  ( 0.000000000000000000, 0.000000000000000000, -1.000000000000000000 ) ) ;
#7294=ORIENTED_EDGE ( 'NONE', *, *, #6168, .T. ) ;
#7302=ORIENTED_EDGE ( 'NONE', *, *, #8983, .T. ) ;
#7314=AXIS2_PLACEMENT_3D ( 'NONE', #7261, #5456, #6566 ) ;
#7316=EDGE_CURVE ( 'NONE', #8705, #8944, #10412, .T. ) ;
#7317=VERTEX_POINT ( 'NONE', #3221 ) ;
#7321=DIRECTION ( 'NONE',  ( 0.000000000000000000, 0.000000000000000000, -1.000000000000000000 ) ) ;
#7335=CARTESIAN_POINT ( 'NONE',  ( -119.9399947101603772, 275.0000000000000000, 35.20508015793608081 ) ) ;
#7343=PLANE ( 'NONE',  #2796 ) ;
#7344=PRODUCT_DEFINITION_FORMATION_WITH_SPECIFIED_SOURCE ( 'ANY', '', #10662, .NOT_KNOWN. ) ;
#7347=DIRECTION ( 'NONE',  ( 0.9595199576812829534, 0.000000000000000000, -0.2816406412634883671 ) ) ;
#7360=ORIENTED_EDGE ( 'NONE', *, *, #4773, .T. ) ;
#7371=ORIENTED_EDGE ( 'NONE', *, *, #5168, .F. ) ;
#7386=CIRCLE ( 'NONE', #9760, 17.00000000000000000 ) ;
#7398=CYLINDRICAL_SURFACE ( 'NONE', #8385, 125.0000000000000284 ) ;
#7407=AXIS2_PLACEMENT_3D ( 'NONE', #2533, #2590, #1724 ) ;
#7418=ORIENTED_EDGE ( 'NONE', *, *, #435, .T. ) ;
#7426=ORIENTED_EDGE ( 'NONE', *, *, #5135, .T. ) ;
#7438=ORIENTED_EDGE ( 'NONE', *, *, #2965, .F. ) ;
#7439=CARTESIAN_POINT ( 'NONE',  ( 97.61745645431939522, 275.0000000000000000, 78.07581056504676553 ) ) ;
#7451=EDGE_LOOP ( 'NONE', ( #6490, #8355, #3689, #6404 ) ) ;
#7458=DIRECTION ( 'NONE',  ( 0.000000000000000000, 0.000000000000000000, 1.000000000000000000 ) ) ;
#7462=CIRCLE ( 'NONE', #2671, 25.00000000000000000 ) ;
#7467=AXIS2_PLACEMENT_3D ( 'NONE', #299, #11717, #6044 ) ;
#7474=VERTEX_POINT ( 'NONE', #11704 ) ;
#7475=CARTESIAN_POINT ( 'NONE',  ( 0.000000000000000000, 75.00000000000001421, -17.00000000000000000 ) ) ;
#7490=CARTESIAN_POINT ( 'NONE',  ( 89.80805993797383735, 275.0000000000000000, 71.82974571984303225 ) ) ;
#7491=CARTESIAN_POINT ( 'NONE',  ( 82.90657655638969459, 275.0000000000000000, 79.06642500897268633 ) ) ;
#7494=EDGE_CURVE ( 'NONE', #6826, #12189, #267, .T. ) ;
#7498=ORIENTED_EDGE ( 'NONE', *, *, #4563, .F. ) ;
#7504=ORIENTED_EDGE ( 'NONE', *, *, #3269, .F. ) ;
#7518=CARTESIAN_POINT ( 'NONE',  ( 0.000000000000000000, 52.00000000000000711, -73.00000000000002842 ) ) ;
#7520=EDGE_CURVE ( 'NONE', #4819, #5619, #654, .T. ) ;
#7553=VECTOR ( 'NONE', #8764, 1000.000000000000000 ) ;
#7562=DIRECTION ( 'NONE',  ( 0.000000000000000000, 0.000000000000000000, 1.000000000000000000 ) ) ;
#7563=DIRECTION ( 'NONE',  ( -0.4999999999999978351, 0.000000000000000000, 0.8660254037844399289 ) ) ;
#7569=ORIENTED_EDGE ( 'NONE', *, *, #10326, .T. ) ;
#7575=CARTESIAN_POINT ( 'NONE',  ( 0.000000000000000000, 52.00000000000000711, 0.000000000000000000 ) ) ;
#7579=AXIS2_PLACEMENT_3D ( 'NONE', #4949, #3950, #8794 ) ;
#7583=ORIENTED_EDGE ( 'NONE', *, *, #11393, .F. ) ;
#7601=ORIENTED_EDGE ( 'NONE', *, *, #9614, .F. ) ;
#7611=ORIENTED_EDGE ( 'NONE', *, *, #7494, .T. ) ;
#7616=DIRECTION ( 'NONE',  ( 0.000000000000000000, 0.000000000000000000, 1.000000000000000000 ) ) ;
#7619=ORIENTED_EDGE ( 'NONE', *, *, #2249, .F. ) ;
#7626=CARTESIAN_POINT ( 'NONE',  ( 0.000000000000000000, 265.0000000000000000, -17.00000000000000000 ) ) ;
#7632=DIRECTION ( 'NONE',  ( 0.000000000000000000, 0.000000000000000000, 1.000000000000000000 ) ) ;
#7635=CARTESIAN_POINT ( 'NONE',  ( 0.000000000000000000, 65.00000000000000000, 0.000000000000000000 ) ) ;
#7637=DIRECTION ( 'NONE',  ( 0.000000000000000000, 1.000000000000000000, 0.000000000000000000 ) ) ;
#7640=AXIS2_PLACEMENT_3D ( 'NONE', #10182, #4391, #12136 ) ;
#7642=ADVANCED_FACE ( 'NONE', ( #2900, #4834 ), #3838, .F. ) ;
#7656=DIRECTION ( 'NONE',  ( 0.000000000000000000, 1.000000000000000000, 0.000000000000000000 ) ) ;
#7658=EDGE_LOOP ( 'NONE', ( #10590, #7078, #5645, #8560 ) ) ;
#7684=FACE_OUTER_BOUND ( 'NONE', #5133, .T. ) ;
#7685=FACE_OUTER_BOUND ( 'NONE', #8918, .T. ) ;
#7693=ORIENTED_EDGE ( 'NONE', *, *, #8127, .T. ) ;
#7702=CARTESIAN_POINT ( 'NONE',  ( 0.000000000000000000, 115.0000000000000142, 0.000000000000000000 ) ) ;
#7710=LINE ( 'NONE', #5785, #2065 ) ;
#7714=ORIENTED_EDGE ( 'NONE', *, *, #5096, .F. ) ;
#7718=ORIENTED_EDGE ( 'NONE', *, *, #7802, .T. ) ;
#7719=FACE_OUTER_BOUND ( 'NONE', #5491, .T. ) ;
#7726=EDGE_CURVE ( 'NONE', #2243, #7094, #8198, .T. ) ;
#7734=VERTEX_POINT ( 'NONE', #146 ) ;
#7738=DIRECTION ( 'NONE',  ( 0.000000000000000000, 1.000000000000000000, 0.000000000000000000 ) ) ;
#7740=DIRECTION ( 'NONE',  ( -0.7236679289129753778, 0.000000000000000000, 0.6901483381584025967 ) ) ;
#7744=DIRECTION ( 'NONE',  ( 0.000000000000000000, 1.000000000000000000, 0.000000000000000000 ) ) ;
#7749=ADVANCED_FACE ( 'NONE', ( #10624 ), #5896, .F. ) ;
#7759=AXIS2_PLACEMENT_3D ( 'NONE', #5610, #9388, #3727 ) ;
#7766=EDGE_CURVE ( 'NONE', #2602, #7317, #4230, .T. ) ;
#7777=CARTESIAN_POINT ( 'NONE',  ( -17.30235457177319347, 275.0000000000000000, -113.6909342308024549 ) ) ;
#7784=ORIENTED_EDGE ( 'NONE', *, *, #10258, .F. ) ;
#7785=CARTESIAN_POINT ( 'NONE',  ( 24.76446302067270722, 275.0000000000000000, -102.0378428393002679 ) ) ;
#7786=LINE ( 'NONE', #1127, #11076 ) ;
#7788=AXIS2_PLACEMENT_3D ( 'NONE', #5880, #11619, #7238 ) ;
#7789=PRODUCT_CONTEXT ( 'NONE', #3181, 'mechanical' ) ;
#7800=ORIENTED_EDGE ( 'NONE', *, *, #8367, .T. ) ;
#7802=EDGE_CURVE ( 'NONE', #1278, #2816, #12209, .T. ) ;
#7811=DIRECTION ( 'NONE',  ( 0.000000000000000000, 0.000000000000000000, -1.000000000000000000 ) ) ;
#7815=VERTEX_POINT ( 'NONE', #8989 ) ;
#7816=ORIENTED_EDGE ( 'NONE', *, *, #2291, .T. ) ;
#7817=DIRECTION ( 'NONE',  ( -0.000000000000000000, -1.000000000000000000, -0.000000000000000000 ) ) ;
#7823=DIRECTION ( 'NONE',  ( 0.000000000000000000, 0.000000000000000000, 1.000000000000000000 ) ) ;
#7844=DIRECTION ( 'NONE',  ( 0.000000000000000000, -0.000000000000000000, 1.000000000000000000 ) ) ;
#7848=ORIENTED_EDGE ( 'NONE', *, *, #3045, .F. ) ;
#7850=CIRCLE ( 'NONE', #2083, 125.0000000000000284 ) ;
#7852=VERTEX_POINT ( 'NONE', #1280 ) ;
#7855=AXIS2_PLACEMENT_3D ( 'NONE', #744, #7288, #4536 ) ;
#7861=CARTESIAN_POINT ( 'NONE',  ( 0.000000000000000000, 75.00000000000001421, -15.00000000000000000 ) ) ;
#7866=ORIENTED_EDGE ( 'NONE', *, *, #9206, .F. ) ;
#7879=DIRECTION ( 'NONE',  ( 0.000000000000000000, 1.000000000000000000, 0.000000000000000000 ) ) ;
#7884=CARTESIAN_POINT ( 'NONE',  ( -116.4243635975518742, 275.0000000000000000, 45.50129185973785440 ) ) ;
#7893=LINE ( 'NONE', #11653, #1408 ) ;
#7898=VERTEX_POINT ( 'NONE', #7932 ) ;
#7902=CARTESIAN_POINT ( 'NONE',  ( 0.000000000000000000, 75.00000000000001421, 25.00000000000000000 ) ) ;
#7904=CARTESIAN_POINT ( 'NONE',  ( 8.939921633775681592E-15, 67.00000000000000000, 73.00000000000002842 ) ) ;
#7925=ORIENTED_EDGE ( 'NONE', *, *, #433, .F. ) ;
#7926=FACE_OUTER_BOUND ( 'NONE', #3192, .T. ) ;
#7928=VERTEX_POINT ( 'NONE', #9048 ) ;
#7932=CARTESIAN_POINT ( 'NONE',  ( -109.9268209223825750, 275.0000000000000000, 32.26598893414599445 ) ) ;
#7937=SURFACE_STYLE_FILL_AREA ( #342 ) ;
#7943=EDGE_CURVE ( 'NONE', #3197, #8944, #651, .T. ) ;
#7959=CARTESIAN_POINT ( 'NONE',  ( 1.836970198721029589E-15, 75.00000000000001421, 15.00000000000000000 ) ) ;
#7969=EDGE_CURVE ( 'NONE', #3197, #4078, #10999, .T. ) ;
#7976=ORIENTED_EDGE ( 'NONE', *, *, #761, .F. ) ;
#7994=DIRECTION ( 'NONE',  ( -0.000000000000000000, -1.000000000000000000, -0.000000000000000000 ) ) ;
#8002=AXIS2_PLACEMENT_3D ( 'NONE', #7635, #1157, #3961 ) ;
#8011=EDGE_CURVE ( 'NONE', #4574, #1744, #4445, .T. ) ;
#8014=ORIENTED_EDGE ( 'NONE', *, *, #8354, .F. ) ;
#8017=EDGE_CURVE ( 'NONE', #1438, #3622, #8070, .T. ) ;
#8019=LINE ( 'NONE', #5170, #3646 ) ;
#8020=ORIENTED_EDGE ( 'NONE', *, *, #2965, .T. ) ;
#8023=ORIENTED_EDGE ( 'NONE', *, *, #9686, .F. ) ;
#8040=CARTESIAN_POINT ( 'NONE',  ( 100.7495955565343451, 285.0000000000000568, 29.57226733266770680 ) ) ;
#8043=LINE ( 'NONE', #8975, #1206 ) ;
#8062=EDGE_LOOP ( 'NONE', ( #8781, #1839 ) ) ;
#8067=CARTESIAN_POINT ( 'NONE',  ( 8.572527594031474570E-15, 65.00000000000000000, 70.00000000000001421 ) ) ;
#8070=CIRCLE ( 'NONE', #6688, 15.00000000000000000 ) ;
#8072=DIRECTION ( 'NONE',  ( 0.000000000000000000, 1.000000000000000000, 0.000000000000000000 ) ) ;
#8079=CARTESIAN_POINT ( 'NONE',  ( 0.000000000000000000, 275.0000000000000000, 0.000000000000000000 ) ) ;
#8082=CYLINDRICAL_SURFACE ( 'NONE', #2464, 100.0000000000000142 ) ;
#8089=DIRECTION ( 'NONE',  ( 0.9595199576812789566, 0.000000000000000000, 0.2816406412635022449 ) ) ;
#8100=DIRECTION ( 'NONE',  ( -0.000000000000000000, -1.000000000000000000, -0.000000000000000000 ) ) ;
#8101=CARTESIAN_POINT ( 'NONE',  ( 6.000000000000000888, 50.00000000000000000, 60.00000000000002132 ) ) ;
#8127=EDGE_CURVE ( 'NONE', #10877, #12351, #5698, .T. ) ;
#8130=FACE_OUTER_BOUND ( 'NONE', #10928, .T. ) ;
#8134=CARTESIAN_POINT ( 'NONE',  ( -27.02024436599226576, 275.0000000000000000, -111.3324139431193345 ) ) ;
#8138=CIRCLE ( 'NONE', #11342, 100.0000000000000142 ) ;
#8139=CIRCLE ( 'NONE', #11942, 73.00000000000002842 ) ;
#8155=ORIENTED_EDGE ( 'NONE', *, *, #10975, .F. ) ;
#8164=VECTOR ( 'NONE', #9948, 1000.000000000000114 ) ;
#8165=ORIENTED_EDGE ( 'NONE', *, *, #1964, .F. ) ;
#8167=AXIS2_PLACEMENT_3D ( 'NONE', #9493, #8688, #9618 ) ;
#8168=ADVANCED_FACE ( 'NONE', ( #176, #9707 ), #1187, .T. ) ;
#8175=CARTESIAN_POINT ( 'NONE',  ( 0.000000000000000000, 75.00000000000001421, 0.000000000000000000 ) ) ;
#8177=FACE_BOUND ( 'NONE', #3492, .T. ) ;
#8180=CARTESIAN_POINT ( 'NONE',  ( 0.000000000000000000, 115.0000000000000142, 0.000000000000000000 ) ) ;
#8181=LINE ( 'NONE', #1649, #3323 ) ;
#8191=DIRECTION ( 'NONE',  ( 0.000000000000000000, 0.000000000000000000, -1.000000000000000000 ) ) ;
#8198=CIRCLE ( 'NONE', #4832, 72.00000000000002842 ) ;
#8199=EDGE_CURVE ( 'NONE', #10214, #4695, #7786, .T. ) ;
#8214=AXIS2_PLACEMENT_3D ( 'NONE', #6346, #10135, #5419 ) ;
#8218=ORIENTED_EDGE ( 'NONE', *, *, #11977, .F. ) ;
#8222=ORIENTED_EDGE ( 'NONE', *, *, #9455, .T. ) ;
#8231=FACE_OUTER_BOUND ( 'NONE', #5860, .T. ) ;
#8233=DIRECTION ( 'NONE',  ( -0.000000000000000000, -1.000000000000000000, -0.000000000000000000 ) ) ;
#8234=CARTESIAN_POINT ( 'NONE',  ( 0.000000000000000000, 260.0000000000000000, 0.000000000000000000 ) ) ;
#8235=TOROIDAL_SURFACE ( 'NONE', #2870, 90.00000000000002842, 10.00000000000000000 ) ;
#8237=CIRCLE ( 'NONE', #4665, 8.000000000000000000 ) ;
#8238=ADVANCED_FACE ( 'NONE', ( #6795 ), #10959, .T. ) ;
#8240=CARTESIAN_POINT ( 'NONE',  ( 0.000000000000000000, 115.0000000000000142, -15.00000000000000000 ) ) ;
#8242=EDGE_CURVE ( 'NONE', #7898, #7852, #9013, .T. ) ;
#8250=EDGE_LOOP ( 'NONE', ( #1117, #8222, #453, #8014, #7504, #9866, #9995 ) ) ;
#8255=AXIS2_PLACEMENT_3D ( 'NONE', #1126, #113, #943 ) ;
#8284=CYLINDRICAL_SURFACE ( 'NONE', #6797, 15.00000000000000000 ) ;
#8292=CARTESIAN_POINT ( 'NONE',  ( 6.000000000000000888, 62.00000000000000000, 60.00000000000002132 ) ) ;
#8293=EDGE_CURVE ( 'NONE', #11519, #7192, #5117, .T. ) ;
#8296=VERTEX_POINT ( 'NONE', #7959 ) ;
#8297=EDGE_CURVE ( 'NONE', #2436, #8994, #1909, .T. ) ;
#8302=CARTESIAN_POINT ( 'NONE',  ( 0.000000000000000000, 50.00000000000000000, 0.000000000000000000 ) ) ;
#8306=DIRECTION ( 'NONE',  ( 0.000000000000000000, 1.000000000000000000, 0.000000000000000000 ) ) ;
#8310=EDGE_LOOP ( 'NONE', ( #7816, #238, #3311, #4386 ) ) ;
#8315=DIRECTION ( 'NONE',  ( 1.000000000000000000, 0.000000000000000000, -0.000000000000000000 ) ) ;
#8320=MECHANICAL_DESIGN_GEOMETRIC_PRESENTATION_REPRESENTATION('',(#356),#6142);
#8330=LINE ( 'NONE', #6594, #2905 ) ;
#8332=CARTESIAN_POINT ( 'NONE',  ( 1.200153863164406345E-14, 265.0000000000000000, 98.00000000000001421 ) ) ;
#8333=DIRECTION ( 'NONE',  ( 0.000000000000000000, 1.000000000000000000, 0.000000000000000000 ) ) ;
#8335=CARTESIAN_POINT ( 'NONE',  ( 0.000000000000000000, 50.00000000000000000, 0.000000000000000000 ) ) ;
#8342=CIRCLE ( 'NONE', #10538, 25.00000000000000000 ) ;
#8347=FACE_OUTER_BOUND ( 'NONE', #3295, .T. ) ;
#8353=VECTOR ( 'NONE', #1268, 1000.000000000000000 ) ;
#8354=EDGE_CURVE ( 'NONE', #7290, #4162, #3908, .T. ) ;
#8355=ORIENTED_EDGE ( 'NONE', *, *, #11393, .T. ) ;
#8358=ORIENTED_EDGE ( 'NONE', *, *, #11281, .T. ) ;
#8361=ORIENTED_EDGE ( 'NONE', *, *, #7250, .F. ) ;
#8362=CIRCLE ( 'NONE', #2395, 105.0000000000000568 ) ;
#8363=VECTOR ( 'NONE', #2270, 1000.000000000000000 ) ;
#8364=CARTESIAN_POINT ( 'NONE',  ( 0.000000000000000000, 275.0000000000000000, 0.000000000000000000 ) ) ;
#8367=EDGE_CURVE ( 'NONE', #6640, #11813, #12073, .T. ) ;
#8368=CARTESIAN_POINT ( 'NONE',  ( -18.80690714323172941, 275.0000000000000000, -123.5771024247852665 ) ) ;
#8370=EDGE_LOOP ( 'NONE', ( #235, #3605, #7240, #6049 ) ) ;
#8375=AXIS2_PLACEMENT_3D ( 'NONE', #10788, #11554, #5131 ) ;
#8377=PLANE ( 'NONE',  #4969 ) ;
#8380=CIRCLE ( 'NONE', #2415, 75.00000000000002842 ) ;
#8381=DIRECTION ( 'NONE',  ( 0.000000000000000000, 1.000000000000000000, 0.000000000000000000 ) ) ;
#8385=AXIS2_PLACEMENT_3D ( 'NONE', #12013, #11268, #599 ) ;
#8386=CIRCLE ( 'NONE', #9983, 25.00000000000000000 ) ;
#8388=ORIENTED_EDGE ( 'NONE', *, *, #10326, .F. ) ;
#8389=CARTESIAN_POINT ( 'NONE',  ( 0.000000000000000000, 52.00000000000000711, -72.00000000000002842 ) ) ;
#8391=LINE ( 'NONE', #12213, #10445 ) ;
#8395=CARTESIAN_POINT ( 'NONE',  ( -27.02024436599226576, 285.0000000000000568, -111.3324139431193345 ) ) ;
#8397=EDGE_CURVE ( 'NONE', #4162, #3178, #8330, .T. ) ;
#8426=DIRECTION ( 'NONE',  ( -0.000000000000000000, -1.000000000000000000, -0.000000000000000000 ) ) ;
#8430=DIRECTION ( 'NONE',  ( 0.000000000000000000, 1.000000000000000000, 0.000000000000000000 ) ) ;
#8435=ORIENTED_EDGE ( 'NONE', *, *, #2291, .F. ) ;
#8447=ORIENTED_EDGE ( 'NONE', *, *, #10707, .T. ) ;
#8451=CARTESIAN_POINT ( 'NONE',  ( 0.000000000000000000, 75.00000000000001421, 0.000000000000000000 ) ) ;
#8454=DIRECTION ( 'NONE',  ( 1.000000000000000000, -0.000000000000000000, 1.224646799147353207E-16 ) ) ;
#8457=VECTOR ( 'NONE', #2851, 1000.000000000000000 ) ;
#8460=ADVANCED_FACE ( 'NONE', ( #99 ), #9632, .T. ) ;
#8464=ORIENTED_EDGE ( 'NONE', *, *, #12103, .F. ) ;
#8483=ORIENTED_EDGE ( 'NONE', *, *, #8367, .F. ) ;
#8495=ADVANCED_FACE ( 'NONE', ( #1477 ), #411, .F. ) ;
#8496=CARTESIAN_POINT ( 'NONE',  ( 116.4243635975512490, 285.0000000000000568, 45.50129185973946733 ) ) ;
#8498=DIRECTION ( 'NONE',  ( 0.000000000000000000, 0.000000000000000000, -1.000000000000000000 ) ) ;
#8503=FACE_OUTER_BOUND ( 'NONE', #6699, .T. ) ;
#8509=EDGE_LOOP ( 'NONE', ( #1738, #9705, #2986, #7718 ) ) ;
#8510=CIRCLE ( 'NONE', #3150, 105.0000000000000426 ) ;
#8517=EDGE_LOOP ( 'NONE', ( #2228, #1878, #11052, #4934 ) ) ;
#8519=VECTOR ( 'NONE', #12137, 1000.000000000000000 ) ;
#8520=ADVANCED_FACE ( 'NONE', ( #4154 ), #4280, .F. ) ;
#8540=EDGE_LOOP ( 'NONE', ( #8877, #11338, #9996, #6291, #11040, #11518 ) ) ;
#8543=ORIENTED_EDGE ( 'NONE', *, *, #926, .F. ) ;
#8550=CIRCLE ( 'NONE', #9138, 100.0000000000000142 ) ;
#8559=CARTESIAN_POINT ( 'NONE',  ( 0.000000000000000000, 115.0000000000000142, 0.000000000000000000 ) ) ;
#8560=ORIENTED_EDGE ( 'NONE', *, *, #2658, .F. ) ;
#8561=DIRECTION ( 'NONE',  ( 0.000000000000000000, 0.000000000000000000, 1.000000000000000000 ) ) ;
#8568=FILL_AREA_STYLE_COLOUR ( '', #10337 ) ;
#8572=CARTESIAN_POINT ( 'NONE',  ( 18.80690714323171164, 285.0000000000000568, -123.5771024247852523 ) ) ;
#8580=DIRECTION ( 'NONE',  ( 1.224646799147352961E-16, 0.000000000000000000, -1.000000000000000000 ) ) ;
#8582=ORIENTED_EDGE ( 'NONE', *, *, #9037, .F. ) ;
#8593=FACE_OUTER_BOUND ( 'NONE', #7658, .T. ) ;
#8600=EDGE_CURVE ( 'NONE', #693, #4574, #1725, .T. ) ;
#8619=VECTOR ( 'NONE', #7347, 1000.000000000000114 ) ;
#8624=DIRECTION ( 'NONE',  ( -0.000000000000000000, -1.000000000000000000, -0.000000000000000000 ) ) ;
#8625=FACE_OUTER_BOUND ( 'NONE', #10598, .T. ) ;
#8631=DIRECTION ( 'NONE',  ( 0.000000000000000000, 0.000000000000000000, 1.000000000000000000 ) ) ;
#8633=CYLINDRICAL_SURFACE ( 'NONE', #419, 9.999999999999994671 ) ;
#8638=DIRECTION ( 'NONE',  ( -0.000000000000000000, -1.000000000000000000, -0.000000000000000000 ) ) ;
#8643=CIRCLE ( 'NONE', #9639, 70.00000000000001421 ) ;
#8644=ORIENTED_EDGE ( 'NONE', *, *, #11532, .T. ) ;
#8664=EDGE_CURVE ( 'NONE', #12219, #5952, #733, .T. ) ;
#8669=CARTESIAN_POINT ( 'NONE',  ( -97.61745645432043261, 285.0000000000000568, 78.07581056504542971 ) ) ;
#8683=ORIENTED_EDGE ( 'NONE', *, *, #8127, .F. ) ;
#8688=DIRECTION ( 'NONE',  ( 0.000000000000000000, 1.000000000000000000, 0.000000000000000000 ) ) ;
#8698=CARTESIAN_POINT ( 'NONE',  ( 18.80690714323171164, 275.0000000000000000, -123.5771024247852523 ) ) ;
#8703=EDGE_CURVE ( 'NONE', #11813, #8705, #1662, .T. ) ;
#8705=VERTEX_POINT ( 'NONE', #6829 ) ;
#8706=DIRECTION ( 'NONE',  ( 0.000000000000000000, 0.000000000000000000, -1.000000000000000000 ) ) ;
#8708=VECTOR ( 'NONE', #6666, 1000.000000000000000 ) ;
#8710=CARTESIAN_POINT ( 'NONE',  ( 0.000000000000000000, 65.00000000000000000, -75.00000000000002842 ) ) ;
#8714=DIRECTION ( 'NONE',  ( -0.7236679289129653858, 0.000000000000000000, -0.6901483381584129218 ) ) ;
#8719=CIRCLE ( 'NONE', #3356, 105.0000000000000426 ) ;
#8734=CARTESIAN_POINT ( 'NONE',  ( 107.1104145097471445, 275.0000000000000000, 41.86118851096031079 ) ) ;
#8738=CIRCLE ( 'NONE', #8167, 105.0000000000000426 ) ;
#8739=VERTEX_POINT ( 'NONE', #5779 ) ;
#8751=EDGE_CURVE ( 'NONE', #12189, #7290, #1036, .T. ) ;
#8764=DIRECTION ( 'NONE',  ( 0.000000000000000000, 1.000000000000000000, 0.000000000000000000 ) ) ;
#8776=ORIENTED_EDGE ( 'NONE', *, *, #3420, .F. ) ;
#8781=ORIENTED_EDGE ( 'NONE', *, *, #1137, .T. ) ;
#8794=DIRECTION ( 'NONE',  ( 0.000000000000000000, 0.000000000000000000, -1.000000000000000000 ) ) ;
#8795=DIRECTION ( 'NONE',  ( 0.000000000000000000, 0.000000000000000000, 1.000000000000000000 ) ) ;
#8797=AXIS2_PLACEMENT_3D ( 'NONE', #5088, #10807, #4083 ) ;
#8807=CARTESIAN_POINT ( 'NONE',  ( 0.000000000000000000, 260.0000000000000000, 0.000000000000000000 ) ) ;
#8810=CARTESIAN_POINT ( 'NONE',  ( 0.000000000000000000, 75.00000000000001421, 0.000000000000000000 ) ) ;
#8814=ADVANCED_FACE ( 'NONE', ( #7073 ), #7133, .T. ) ;
#8819=AXIS2_PLACEMENT_3D ( 'NONE', #10247, #10185, #6525 ) ;
#8820=CIRCLE ( 'NONE', #675, 98.00000000000001421 ) ;
#8825=CYLINDRICAL_SURFACE ( 'NONE', #10144, 100.0000000000000284 ) ;
#8829=VECTOR ( 'NONE', #2166, 1000.000000000000000 ) ;
#8830=ORIENTED_EDGE ( 'NONE', *, *, #4479, .T. ) ;
#8848=PLANE ( 'NONE',  #12076 ) ;
#8853=ORIENTED_EDGE ( 'NONE', *, *, #2249, .T. ) ;
#8855=EDGE_CURVE ( 'NONE', #3002, #10848, #526, .T. ) ;
#8861=AXIS2_PLACEMENT_3D ( 'NONE', #4347, #12029, #5357 ) ;
#8862=ORIENTED_EDGE ( 'NONE', *, *, #11148, .F. ) ;
#8868=ORIENTED_EDGE ( 'NONE', *, *, #7520, .F. ) ;
#8870=DIRECTION ( 'NONE',  ( 0.000000000000000000, 0.000000000000000000, 1.000000000000000000 ) ) ;
#8877=ORIENTED_EDGE ( 'NONE', *, *, #7943, .F. ) ;
#8883=DIRECTION ( 'NONE',  ( -0.6901483381584025967, 0.000000000000000000, -0.7236679289129753778 ) ) ;
#8884=EDGE_CURVE ( 'NONE', #693, #3178, #7013, .T. ) ;
#8888=DIRECTION ( 'NONE',  ( 0.8660254037844362651, 0.000000000000000000, 0.5000000000000039968 ) ) ;
#8892=DIRECTION ( 'NONE',  ( -0.000000000000000000, -1.000000000000000000, -0.000000000000000000 ) ) ;
#8910=ORIENTED_EDGE ( 'NONE', *, *, #10258, .T. ) ;
#8912=CARTESIAN_POINT ( 'NONE',  ( 0.000000000000000000, 285.0000000000000568, 0.000000000000000000 ) ) ;
#8918=EDGE_LOOP ( 'NONE', ( #6193, #479, #6064, #5044, #8483, #11550 ) ) ;
#8922=ADVANCED_FACE ( 'NONE', ( #585 ), #10174, .T. ) ;
#8944=VERTEX_POINT ( 'NONE', #11124 ) ;
#8949=ORIENTED_EDGE ( 'NONE', *, *, #8293, .F. ) ;
#8951=DIRECTION ( 'NONE',  ( 0.000000000000000000, 0.000000000000000000, 1.000000000000000000 ) ) ;
#8963=CARTESIAN_POINT ( 'NONE',  ( 1.224646799147353533E-14, 285.0000000000000568, -100.0000000000000284 ) ) ;
#8965=EDGE_CURVE ( 'NONE', #7898, #2259, #8181, .T. ) ;
#8970=EDGE_LOOP ( 'NONE', ( #11497, #6732 ) ) ;
#8975=CARTESIAN_POINT ( 'NONE',  ( 82.90657655638969459, 275.0000000000000000, 79.06642500897268633 ) ) ;
#8978=ADVANCED_BREP_SHAPE_REPRESENTATION ( '', ( #461, #1612 ), #1360 ) ;
#8979=VECTOR ( 'NONE', #54, 1000.000000000000000 ) ;
#8982=DIRECTION ( 'NONE',  ( 0.000000000000000000, 1.000000000000000000, 0.000000000000000000 ) ) ;
#8983=EDGE_CURVE ( 'NONE', #5612, #12245, #1535, .T. ) ;
#8986=DIRECTION ( 'NONE',  ( 0.000000000000000000, 0.000000000000000000, 1.000000000000000000 ) ) ;
#8989=CARTESIAN_POINT ( 'NONE',  ( 0.000000000000000000, 65.00000000000000000, 25.00000000000000000 ) ) ;
#8992=ORIENTED_EDGE ( 'NONE', *, *, #7034, .F. ) ;
#8994=VERTEX_POINT ( 'NONE', #11252 ) ;
#8999=DIRECTION ( 'NONE',  ( -0.000000000000000000, -1.000000000000000000, -0.000000000000000000 ) ) ;
#9010=FACE_OUTER_BOUND ( 'NONE', #6180, .T. ) ;
#9012=DIRECTION ( 'NONE',  ( 0.000000000000000000, 0.000000000000000000, 1.000000000000000000 ) ) ;
#9013=LINE ( 'NONE', #10019, #4094 ) ;
#9015=DIRECTION ( 'NONE',  ( 1.224646799147351482E-16, 0.000000000000000000, -1.000000000000000000 ) ) ;
#9018=ORIENTED_EDGE ( 'NONE', *, *, #9794, .F. ) ;
#9023=EDGE_CURVE ( 'NONE', #1518, #5644, #10688, .T. ) ;
#9037=EDGE_CURVE ( 'NONE', #108, #1744, #12289, .T. ) ;
#9048=CARTESIAN_POINT ( 'NONE',  ( -5.999999999999999112, 50.00000000000000000, 60.00000000000002132 ) ) ;
#9054=EDGE_CURVE ( 'NONE', #9195, #3744, #4632, .T. ) ;
#9056=( NAMED_UNIT ( * ) PLANE_ANGLE_UNIT ( ) SI_UNIT ( $, .RADIAN. ) );
#9058=AXIS2_PLACEMENT_3D ( 'NONE', #6120, #9971, #6179 ) ;
#9060=CARTESIAN_POINT ( 'NONE',  ( 8.817456953860944867E-15, 67.00000000000000000, 72.00000000000002842 ) ) ;
#9061=DIRECTION ( 'NONE',  ( 0.000000000000000000, -0.000000000000000000, 1.000000000000000000 ) ) ;
#9064=DIRECTION ( 'NONE',  ( -0.000000000000000000, -1.000000000000000000, -0.000000000000000000 ) ) ;
#9068=CARTESIAN_POINT ( 'NONE',  ( 90.45849111412074706, 275.0000000000000000, 86.26854226980164242 ) ) ;
#9069=AXIS2_PLACEMENT_3D ( 'NONE', #4218, #6962, #4333 ) ;
#9071=DIRECTION ( 'NONE',  ( -0.000000000000000000, -1.000000000000000000, -0.000000000000000000 ) ) ;
#9075=DIRECTION ( 'NONE',  ( -1.000000000000000000, 0.000000000000000000, 0.000000000000000000 ) ) ;
#9076=ORIENTED_EDGE ( 'NONE', *, *, #1595, .F. ) ;
#9087=VERTEX_POINT ( 'NONE', #71 ) ;
#9102=ORIENTED_EDGE ( 'NONE', *, *, #368, .F. ) ;
#9103=PLANE ( 'NONE',  #1090 ) ;
#9105=ORIENTED_EDGE ( 'NONE', *, *, #8011, .T. ) ;
#9114=UNCERTAINTY_MEASURE_WITH_UNIT (LENGTH_MEASURE( 1.000000000000000082E-05 ), #3339, 'distance_accuracy_value', 'NONE');
#9115=CYLINDRICAL_SURFACE ( 'NONE', #7640, 72.00000000000002842 ) ;
#9117=ADVANCED_FACE ( 'NONE', ( #7684 ), #11889, .T. ) ;
#9119=FACE_OUTER_BOUND ( 'NONE', #8370, .T. ) ;
#9129=CYLINDRICAL_SURFACE ( 'NONE', #9378, 9.999999999999994671 ) ;
#9136=CIRCLE ( 'NONE', #3775, 70.00000000000001421 ) ;
#9138=AXIS2_PLACEMENT_3D ( 'NONE', #10614, #9669, #1148 ) ;
#9141=LINE ( 'NONE', #6171, #10349 ) ;
#9150=CARTESIAN_POINT ( 'NONE',  ( -18.80690714323172941, 285.0000000000000568, -123.5771024247852665 ) ) ;
#9153=CARTESIAN_POINT ( 'NONE',  ( 0.000000000000000000, 67.00000000000000000, 0.000000000000000000 ) ) ;
#9166=ORIENTED_EDGE ( 'NONE', *, *, #10820, .T. ) ;
#9171=DIRECTION ( 'NONE',  ( -0.000000000000000000, -1.000000000000000000, -0.000000000000000000 ) ) ;
#9179=EDGE_CURVE ( 'NONE', #5710, #7734, #6692, .T. ) ;
#9184=FACE_OUTER_BOUND ( 'NONE', #3732, .T. ) ;
#9195=VERTEX_POINT ( 'NONE', #6877 ) ;
#9206=EDGE_CURVE ( 'NONE', #9781, #7928, #1326, .T. ) ;
#9208=ORIENTED_EDGE ( 'NONE', *, *, #89, .F. ) ;
#9222=CARTESIAN_POINT ( 'NONE',  ( 1.224646799147353533E-14, 260.0000000000000000, -100.0000000000000284 ) ) ;
#9225=DIRECTION ( 'NONE',  ( 0.000000000000000000, 1.000000000000000000, 0.000000000000000000 ) ) ;
#9230=DIRECTION ( 'NONE',  ( 0.000000000000000000, 1.000000000000000000, 0.000000000000000000 ) ) ;
#9238=EDGE_CURVE ( 'NONE', #3744, #7474, #2129, .T. ) ;
#9245=CARTESIAN_POINT ( 'NONE',  ( 0.000000000000000000, 75.00000000000001421, 90.00000000000002842 ) ) ;
#9248=CIRCLE ( 'NONE', #7044, 90.00000000000002842 ) ;
#9257=CLOSED_SHELL ( 'NONE', ( #2257, #1446, #12021, #1358, #1988, #4076, #1121, #729, #10056, #4964, #4446, #10380, #3966, #8922, #1681, #7006, #253, #7749, #2214, #1125, #10166, #12046, #7642, #4937, #6103, #1105, #9117, #8168, #5110, #5704, #3920, #2037, #8495, #4526, #4295, #3358, #8814, #2334, #6230, #5821, #3833, #1973, #6849, #5446, #9715, #1711, #8520, #1987, #4845, #5287, #10821, #12034, #92, #12224, #9581, #8460, #6080, #8238, #527, #9745, #3860, #2036 ) ) ;
#9269=VERTEX_POINT ( 'NONE', #11867 ) ;
#9270=CARTESIAN_POINT ( 'NONE',  ( -24.76446302067273209, 275.0000000000000000, -102.0378428393002679 ) ) ;
#9273=DIRECTION ( 'NONE',  ( 0.000000000000000000, 0.000000000000000000, 1.000000000000000000 ) ) ;
#9277=DIRECTION ( 'NONE',  ( 0.000000000000000000, 1.000000000000000000, 0.000000000000000000 ) ) ;
#9284=DIRECTION ( 'NONE',  ( 0.000000000000000000, -1.000000000000000000, 0.000000000000000000 ) ) ;
#9288=DIRECTION ( 'NONE',  ( -0.000000000000000000, -1.000000000000000000, -0.000000000000000000 ) ) ;
#9301=ORIENTED_EDGE ( 'NONE', *, *, #8751, .F. ) ;
#9307=DIRECTION ( 'NONE',  ( 0.000000000000000000, 1.000000000000000000, 0.000000000000000000 ) ) ;
#9309=EDGE_CURVE ( 'NONE', #9087, #4827, #11682, .T. ) ;
#9332=VECTOR ( 'NONE', #8089, 1000.000000000000000 ) ;
#9364=CIRCLE ( 'NONE', #612, 73.00000000000002842 ) ;
#9365=CIRCLE ( 'NONE', #10369, 15.00000000000000000 ) ;
#9372=CARTESIAN_POINT ( 'NONE',  ( 116.4243635975512490, 275.0000000000000000, 45.50129185973946733 ) ) ;
#9378=AXIS2_PLACEMENT_3D ( 'NONE', #12022, #12210, #3477 ) ;
#9379=CARTESIAN_POINT ( 'NONE',  ( 0.000000000000000000, 65.00000000000000000, 0.000000000000000000 ) ) ;
#9380=PLANE ( 'NONE',  #1898 ) ;
#9384=DIRECTION ( 'NONE',  ( 0.000000000000000000, 1.000000000000000000, 0.000000000000000000 ) ) ;
#9386=CARTESIAN_POINT ( 'NONE',  ( 3.061616997868383043E-15, 75.00000000000001421, -25.00000000000000000 ) ) ;
#9388=DIRECTION ( 'NONE',  ( 0.000000000000000000, 1.000000000000000000, 0.000000000000000000 ) ) ;
#9392=ORIENTED_EDGE ( 'NONE', *, *, #9023, .T. ) ;
#9398=ORIENTED_EDGE ( 'NONE', *, *, #6788, .F. ) ;
#9409=ORIENTED_EDGE ( 'NONE', *, *, #11893, .F. ) ;
#9427=DIRECTION ( 'NONE',  ( 0.000000000000000000, -0.000000000000000000, 1.000000000000000000 ) ) ;
#9432=LINE ( 'NONE', #3841, #11994 ) ;
#9433=EDGE_CURVE ( 'NONE', #4433, #5644, #11990, .T. ) ;
#9436=CARTESIAN_POINT ( 'NONE',  ( 0.000000000000000000, 275.0000000000000000, 0.000000000000000000 ) ) ;
#9455=EDGE_CURVE ( 'NONE', #1744, #5680, #2032, .T. ) ;
#9458=LINE ( 'NONE', #4859, #8708 ) ;
#9477=ORIENTED_EDGE ( 'NONE', *, *, #6484, .T. ) ;
#9484=AXIS2_PLACEMENT_3D ( 'NONE', #8912, #9724, #6182 ) ;
#9492=DIRECTION ( 'NONE',  ( 0.000000000000000000, 1.000000000000000000, 0.000000000000000000 ) ) ;
#9493=CARTESIAN_POINT ( 'NONE',  ( 0.000000000000000000, 285.0000000000000568, 0.000000000000000000 ) ) ;
#9502=EDGE_LOOP ( 'NONE', ( #1525, #8830, #4227, #5435 ) ) ;
#9504=CARTESIAN_POINT ( 'NONE',  ( 0.000000000000000000, 65.00000000000000000, 0.000000000000000000 ) ) ;
#9505=DIRECTION ( 'NONE',  ( 0.000000000000000000, 0.000000000000000000, 1.000000000000000000 ) ) ;
#9515=EDGE_CURVE ( 'NONE', #5710, #10706, #6613, .T. ) ;
#9521=DIRECTION ( 'NONE',  ( 0.000000000000000000, 0.000000000000000000, 1.000000000000000000 ) ) ;
#9543=CARTESIAN_POINT ( 'NONE',  ( 0.000000000000000000, 285.0000000000000568, 0.000000000000000000 ) ) ;
#9544=VECTOR ( 'NONE', #572, 1000.000000000000000 ) ;
#9553=PRODUCT_DEFINITION_SHAPE ( 'NONE', 'NONE',  #5201 ) ;
#9559=CARTESIAN_POINT ( 'NONE',  ( -6.000000000000000000, 65.00000000000000000, 69.74238309665079782 ) ) ;
#9562=CARTESIAN_POINT ( 'NONE',  ( 0.000000000000000000, 0.000000000000000000, 0.000000000000000000 ) ) ;
#9564=EDGE_CURVE ( 'NONE', #544, #8739, #119, .T. ) ;
#9579=AXIS2_PLACEMENT_3D ( 'NONE', #5503, #9284, #765 ) ;
#9581=ADVANCED_FACE ( 'NONE', ( #8593 ), #1869, .T. ) ;
#9585=ORIENTED_EDGE ( 'NONE', *, *, #7316, .T. ) ;
#9586=CARTESIAN_POINT ( 'NONE',  ( 89.80805993797383735, 285.0000000000000568, 81.82974571984303225 ) ) ;
#9590=CARTESIAN_POINT ( 'NONE',  ( -75.98513253586240523, 275.0000000000000000, 72.46557550663233371 ) ) ;
#9614=EDGE_CURVE ( 'NONE', #12345, #10879, #7204, .T. ) ;
#9618=DIRECTION ( 'NONE',  ( 0.000000000000000000, 0.000000000000000000, 1.000000000000000000 ) ) ;
#9621=ORIENTED_EDGE ( 'NONE', *, *, #4468, .T. ) ;
#9622=CIRCLE ( 'NONE', #5263, 72.00000000000002842 ) ;
#9625=ORIENTED_EDGE ( 'NONE', *, *, #2062, .T. ) ;
#9632=CYLINDRICAL_SURFACE ( 'NONE', #9858, 10.00000000000000178 ) ;
#9637=FACE_OUTER_BOUND ( 'NONE', #8540, .T. ) ;
#9639=AXIS2_PLACEMENT_3D ( 'NONE', #11493, #3005, #1258 ) ;
#9651=DIRECTION ( 'NONE',  ( 0.000000000000000000, 1.000000000000000000, 0.000000000000000000 ) ) ;
#9652=EDGE_LOOP ( 'NONE', ( #2673, #7976, #7583, #1789 ) ) ;
#9655=CIRCLE ( 'NONE', #4100, 100.0000000000000284 ) ;
#9669=DIRECTION ( 'NONE',  ( 0.000000000000000000, 1.000000000000000000, 0.000000000000000000 ) ) ;
#9672=AXIS2_PLACEMENT_3D ( 'NONE', #4707, #8381, #12204 ) ;
#9680=LINE ( 'NONE', #3026, #8363 ) ;
#9686=EDGE_CURVE ( 'NONE', #2386, #7815, #8386, .T. ) ;
#9691=CARTESIAN_POINT ( 'NONE',  ( 0.000000000000000000, 50.00000000000000000, 0.000000000000000000 ) ) ;
#9694=CARTESIAN_POINT ( 'NONE',  ( 0.000000000000000000, 265.0000000000000000, -15.00000000000000000 ) ) ;
#9701=AXIS2_PLACEMENT_3D ( 'NONE', #12164, #3493, #11224 ) ;
#9703=CARTESIAN_POINT ( 'NONE',  ( 1.224646799147353375E-14, 260.0000000000000000, 100.0000000000000142 ) ) ;
#9704=CARTESIAN_POINT ( 'NONE',  ( -18.80690714323172941, 275.0000000000000000, -123.5771024247852665 ) ) ;
#9705=ORIENTED_EDGE ( 'NONE', *, *, #7166, .F. ) ;
#9706=CARTESIAN_POINT ( 'NONE',  ( 6.000000000000000000, 65.00000000000000000, 69.74238309665078361 ) ) ;
#9707=FACE_BOUND ( 'NONE', #8970, .T. ) ;
#9715=ADVANCED_FACE ( 'NONE', ( #5417 ), #9129, .T. ) ;
#9724=DIRECTION ( 'NONE',  ( -0.000000000000000000, -1.000000000000000000, -0.000000000000000000 ) ) ;
#9733=ORIENTED_EDGE ( 'NONE', *, *, #3034, .T. ) ;
#9734=ORIENTED_EDGE ( 'NONE', *, *, #7040, .F. ) ;
#9743=DIRECTION ( 'NONE',  ( 0.000000000000000000, 0.000000000000000000, -1.000000000000000000 ) ) ;
#9745=ADVANCED_FACE ( 'NONE', ( #603 ), #1542, .T. ) ;
#9748=CARTESIAN_POINT ( 'NONE',  ( 0.000000000000000000, 50.00000000000000000, -75.00000000000002842 ) ) ;
#9752=LINE ( 'NONE', #2159, #3765 ) ;
#9760=AXIS2_PLACEMENT_3D ( 'NONE', #4204, #7994, #4263 ) ;
#9781=VERTEX_POINT ( 'NONE', #10123 ) ;
#9784=ORIENTED_EDGE ( 'NONE', *, *, #8397, .T. ) ;
#9794=EDGE_CURVE ( 'NONE', #1438, #8296, #2406, .T. ) ;
#9799=DIRECTION ( 'NONE',  ( 0.000000000000000000, -0.000000000000000000, 1.000000000000000000 ) ) ;
#9837=CIRCLE ( 'NONE', #88, 105.0000000000000426 ) ;
#9844=CIRCLE ( 'NONE', #6082, 15.00000000000000000 ) ;
#9850=CYLINDRICAL_SURFACE ( 'NONE', #6483, 73.00000000000002842 ) ;
#9858=AXIS2_PLACEMENT_3D ( 'NONE', #6031, #8072, #1541 ) ;
#9866=ORIENTED_EDGE ( 'NONE', *, *, #7228, .T. ) ;
#9870=DIRECTION ( 'NONE',  ( -0.2358520287683116834, 0.000000000000000000, 0.9717889794219068955 ) ) ;
#9871=DIRECTION ( 'NONE',  ( -0.000000000000000000, -1.000000000000000000, -0.000000000000000000 ) ) ;
#9873=EDGE_CURVE ( 'NONE', #5952, #12219, #11791, .T. ) ;
#9892=VERTEX_POINT ( 'NONE', #7518 ) ;
#9902=EDGE_CURVE ( 'NONE', #7192, #7928, #9432, .T. ) ;
#9912=LINE ( 'NONE', #11805, #7274 ) ;
#9921=DIRECTION ( 'NONE',  ( 0.000000000000000000, 0.000000000000000000, 1.000000000000000000 ) ) ;
#9935=DIRECTION ( 'NONE',  ( -0.000000000000000000, -1.000000000000000000, -0.000000000000000000 ) ) ;
#9948=DIRECTION ( 'NONE',  ( -0.7236679289129653858, 0.000000000000000000, -0.6901483381584129218 ) ) ;
#9954=AXIS2_PLACEMENT_3D ( 'NONE', #523, #7132, #8795 ) ;
#9966=CIRCLE ( 'NONE', #10569, 10.00000000000000178 ) ;
#9971=DIRECTION ( 'NONE',  ( 0.000000000000000000, 1.000000000000000000, 0.000000000000000000 ) ) ;
#9983=AXIS2_PLACEMENT_3D ( 'NONE', #9379, #672, #4653 ) ;
#9992=CARTESIAN_POINT ( 'NONE',  ( 3.061616997868383043E-15, 65.00000000000000000, -25.00000000000000000 ) ) ;
#9995=ORIENTED_EDGE ( 'NONE', *, *, #11977, .T. ) ;
#9996=ORIENTED_EDGE ( 'NONE', *, *, #5332, .T. ) ;
#10004=EDGE_CURVE ( 'NONE', #8739, #5619, #1800, .T. ) ;
#10005=CARTESIAN_POINT ( 'NONE',  ( 0.000000000000000000, 275.0000000000000000, 0.000000000000000000 ) ) ;
#10012=CARTESIAN_POINT ( 'NONE',  ( 90.45849111412074706, 275.0000000000000000, 86.26854226980164242 ) ) ;
#10013=CARTESIAN_POINT ( 'NONE',  ( 89.80805993797383735, 275.0000000000000000, 81.82974571984303225 ) ) ;
#10019=CARTESIAN_POINT ( 'NONE',  ( -119.9399947101603772, 275.0000000000000000, 35.20508015793608081 ) ) ;
#10034=DIRECTION ( 'NONE',  ( 0.9717889794219071176, 0.000000000000000000, -0.2358520287683112393 ) ) ;
#10050=ORIENTED_EDGE ( 'NONE', *, *, #2156, .T. ) ;
#10054=AXIS2_PLACEMENT_3D ( 'NONE', #7335, #793, #11952 ) ;
#10056=ADVANCED_FACE ( 'NONE', ( #5959 ), #3088, .F. ) ;
#10080=DIRECTION ( 'NONE',  ( 1.224646799147353454E-16, 0.000000000000000000, -1.000000000000000000 ) ) ;
#10081=LINE ( 'NONE', #7039, #9332 ) ;
#10111=CIRCLE ( 'NONE', #4747, 25.00000000000000000 ) ;
#10123=CARTESIAN_POINT ( 'NONE',  ( 6.000000000000000888, 50.00000000000000000, 60.00000000000002132 ) ) ;
#10132=COLOUR_RGB ( '', 0.09019608, 0.27058824, 0.51372549) ;
#10135=DIRECTION ( 'NONE',  ( 0.000000000000000000, 1.000000000000000000, 0.000000000000000000 ) ) ;
#10141=ORIENTED_EDGE ( 'NONE', *, *, #9206, .T. ) ;
#10144=AXIS2_PLACEMENT_3D ( 'NONE', #10644, #3923, #2924 ) ;
#10145=ORIENTED_EDGE ( 'NONE', *, *, #3601, .T. ) ;
#10158=DIRECTION ( 'NONE',  ( -0.2358520287683112115, 0.000000000000000000, -0.9717889794219070065 ) ) ;
#10166=ADVANCED_FACE ( 'NONE', ( #460 ), #4265, .T. ) ;
#10174=CYLINDRICAL_SURFACE ( 'NONE', #7314, 17.00000000000000000 ) ;
#10182=CARTESIAN_POINT ( 'NONE',  ( 0.000000000000000000, 65.00000000000000000, 0.000000000000000000 ) ) ;
#10185=DIRECTION ( 'NONE',  ( 0.000000000000000000, 1.000000000000000000, 0.000000000000000000 ) ) ;
#10186=DIRECTION ( 'NONE',  ( 0.000000000000000000, 1.000000000000000000, 0.000000000000000000 ) ) ;
#10201=DIRECTION ( 'NONE',  ( 0.000000000000000000, 1.000000000000000000, 0.000000000000000000 ) ) ;
#10203=AXIS2_PLACEMENT_3D ( 'NONE', #1440, #10846, #5129 ) ;
#10208=DIRECTION ( 'NONE',  ( 1.000000000000000000, 0.000000000000000000, -1.065814103640150437E-14 ) ) ;
#10209=AXIS2_PLACEMENT_3D ( 'NONE', #9691, #1167, #2161 ) ;
#10214=VERTEX_POINT ( 'NONE', #10424 ) ;
#10215=CARTESIAN_POINT ( 'NONE',  ( 0.000000000000000000, 265.0000000000000000, 0.000000000000000000 ) ) ;
#10218=DIRECTION ( 'NONE',  ( 0.000000000000000000, 0.000000000000000000, 1.000000000000000000 ) ) ;
#10222=AXIS2_PLACEMENT_3D ( 'NONE', #10284, #5562, #10218 ) ;
#10241=ORIENTED_EDGE ( 'NONE', *, *, #5546, .T. ) ;
#10247=CARTESIAN_POINT ( 'NONE',  ( 0.000000000000000000, 260.0000000000000000, 0.000000000000000000 ) ) ;
#10248=AXIS2_PLACEMENT_3D ( 'NONE', #11681, #4070, #2014 ) ;
#10249=DIRECTION ( 'NONE',  ( 0.000000000000000000, 1.000000000000000000, 0.000000000000000000 ) ) ;
#10258=EDGE_CURVE ( 'NONE', #3401, #5298, #6189, .T. ) ;
#10262=ORIENTED_EDGE ( 'NONE', *, *, #11516, .T. ) ;
#10267=FACE_OUTER_BOUND ( 'NONE', #441, .T. ) ;
#10278=EDGE_LOOP ( 'NONE', ( #11227, #7302, #10241, #1742 ) ) ;
#10282=ORIENTED_EDGE ( 'NONE', *, *, #433, .T. ) ;
#10284=CARTESIAN_POINT ( 'NONE',  ( 0.000000000000000000, 115.0000000000000142, 0.000000000000000000 ) ) ;
#10326=EDGE_CURVE ( 'NONE', #10848, #3002, #9364, .T. ) ;
#10335=ORIENTED_EDGE ( 'NONE', *, *, #4479, .F. ) ;
#10337=COLOUR_RGB ( '', 0.09019608, 0.27058824, 0.51372549) ;
#10349=VECTOR ( 'NONE', #12036, 1000.000000000000000 ) ;
#10350=APPLICATION_CONTEXT ( 'automotive_design' ) ;
#10362=AXIS2_PLACEMENT_3D ( 'NONE', #5465, #12263, #6642 ) ;
#10366=DIRECTION ( 'NONE',  ( 0.000000000000000000, 0.000000000000000000, 1.000000000000000000 ) ) ;
#10369=AXIS2_PLACEMENT_3D ( 'NONE', #830, #9288, #12300 ) ;
#10370=CARTESIAN_POINT ( 'NONE',  ( 29.48150359603894088, 275.0000000000000000, -121.4736224277384053 ) ) ;
#10374=FACE_OUTER_BOUND ( 'NONE', #5235, .T. ) ;
#10380=ADVANCED_FACE ( 'NONE', ( #7685 ), #1147, .F. ) ;
#10396=DIRECTION ( 'NONE',  ( 1.000000000000000000, 0.000000000000000000, 0.000000000000000000 ) ) ;
#10412=CIRCLE ( 'NONE', #465, 70.00000000000001421 ) ;
#10418=ORIENTED_EDGE ( 'NONE', *, *, #2734, .F. ) ;
#10422=ORIENTED_EDGE ( 'NONE', *, *, #1137, .F. ) ;
#10424=CARTESIAN_POINT ( 'NONE',  ( 82.90657655638969459, 285.0000000000000568, 79.06642500897268633 ) ) ;
#10429=ORIENTED_EDGE ( 'NONE', *, *, #2513, .F. ) ;
#10434=ORIENTED_EDGE ( 'NONE', *, *, #6196, .F. ) ;
#10435=DIRECTION ( 'NONE',  ( 0.000000000000000000, 1.000000000000000000, 0.000000000000000000 ) ) ;
#10445=VECTOR ( 'NONE', #3425, 1000.000000000000000 ) ;
#10462=DIRECTION ( 'NONE',  ( 0.000000000000000000, 0.000000000000000000, 1.000000000000000000 ) ) ;
#10464=CIRCLE ( 'NONE', #5101, 72.00000000000002842 ) ;
#10466=EDGE_LOOP ( 'NONE', ( #10755, #3315 ) ) ;
#10468=FACE_OUTER_BOUND ( 'NONE', #5853, .T. ) ;
#10476=CARTESIAN_POINT ( 'NONE',  ( 0.000000000000000000, 275.0000000000000000, 0.000000000000000000 ) ) ;
#10508=EDGE_CURVE ( 'NONE', #5250, #10877, #5253, .T. ) ;
#10510=( NAMED_UNIT ( * ) SI_UNIT ( $, .STERADIAN. ) SOLID_ANGLE_UNIT ( ) );
#10538=AXIS2_PLACEMENT_3D ( 'NONE', #2694, #9225, #3631 ) ;
#10539=ORIENTED_EDGE ( 'NONE', *, *, #11516, .F. ) ;
#10550=CIRCLE ( 'NONE', #12161, 125.0000000000000284 ) ;
#10551=LINE ( 'NONE', #7626, #4181 ) ;
#10557=AXIS2_PLACEMENT_3D ( 'NONE', #2091, #10749, #8870 ) ;
#10567=DIRECTION ( 'NONE',  ( 0.000000000000000000, 1.000000000000000000, 0.000000000000000000 ) ) ;
#10569=AXIS2_PLACEMENT_3D ( 'NONE', #11103, #502, #439 ) ;
#10584=CYLINDRICAL_SURFACE ( 'NONE', #2599, 125.0000000000000284 ) ;
#10590=ORIENTED_EDGE ( 'NONE', *, *, #12178, .F. ) ;
#10598=EDGE_LOOP ( 'NONE', ( #4644, #7109, #10840, #8435 ) ) ;
#10604=CARTESIAN_POINT ( 'NONE',  ( 0.000000000000000000, 275.0000000000000000, 0.000000000000000000 ) ) ;
#10614=CARTESIAN_POINT ( 'NONE',  ( 0.000000000000000000, 75.00000000000001421, 0.000000000000000000 ) ) ;
#10622=DIRECTION ( 'NONE',  ( 0.000000000000000000, 1.000000000000000000, 0.000000000000000000 ) ) ;
#10624=FACE_OUTER_BOUND ( 'NONE', #11785, .T. ) ;
#10630=AXIS2_PLACEMENT_3D ( 'NONE', #7902, #5056, #491 ) ;
#10639=VERTEX_POINT ( 'NONE', #7491 ) ;
#10644=CARTESIAN_POINT ( 'NONE',  ( 0.000000000000000000, 260.0000000000000000, 0.000000000000000000 ) ) ;
#10662=PRODUCT ( 'Clear Processing Bowl', 'Clear Processing Bowl', '', ( #7789 ) ) ;
#10685=VERTEX_POINT ( 'NONE', #699 ) ;
#10688=CIRCLE ( 'NONE', #4312, 9.999999999999994671 ) ;
#10694=DIRECTION ( 'NONE',  ( 1.224646799147352961E-16, 0.000000000000000000, -1.000000000000000000 ) ) ;
#10702=FACE_OUTER_BOUND ( 'NONE', #6501, .T. ) ;
#10706=VERTEX_POINT ( 'NONE', #1755 ) ;
#10707=EDGE_CURVE ( 'NONE', #5644, #6060, #11302, .T. ) ;
#10709=CARTESIAN_POINT ( 'NONE',  ( 89.80805993797383735, 285.0000000000000568, 71.82974571984303225 ) ) ;
#10713=DIRECTION ( 'NONE',  ( 0.000000000000000000, 1.000000000000000000, 0.000000000000000000 ) ) ;
#10715=DIRECTION ( 'NONE',  ( -0.000000000000000000, -1.000000000000000000, -0.000000000000000000 ) ) ;
#10731=DIRECTION ( 'NONE',  ( -1.000000000000000000, 0.000000000000000000, 0.000000000000000000 ) ) ;
#10749=DIRECTION ( 'NONE',  ( 0.000000000000000000, 1.000000000000000000, 0.000000000000000000 ) ) ;
#10754=( NAMED_UNIT ( * ) PLANE_ANGLE_UNIT ( ) SI_UNIT ( $, .RADIAN. ) );
#10755=ORIENTED_EDGE ( 'NONE', *, *, #89, .T. ) ;
#10788=CARTESIAN_POINT ( 'NONE',  ( 0.000000000000000000, 260.0000000000000000, 0.000000000000000000 ) ) ;
#10803=DIRECTION ( 'NONE',  ( 0.000000000000000000, 0.000000000000000000, 1.000000000000000000 ) ) ;
#10807=DIRECTION ( 'NONE',  ( 0.000000000000000000, 1.000000000000000000, 0.000000000000000000 ) ) ;
#10820=EDGE_CURVE ( 'NONE', #5250, #1500, #8380, .T. ) ;
#10821=ADVANCED_FACE ( 'NONE', ( #6861 ), #1008, .F. ) ;
#10823=VECTOR ( 'NONE', #10715, 1000.000000000000000 ) ;
#10839=TOROIDAL_SURFACE ( 'NONE', #7855, 90.00000000000002842, 10.00000000000000000 ) ;
#10840=ORIENTED_EDGE ( 'NONE', *, *, #368, .T. ) ;
#10842=CIRCLE ( 'NONE', #4883, 125.0000000000000568 ) ;
#10845=CARTESIAN_POINT ( 'NONE',  ( 107.1104145097471445, 285.0000000000000568, 41.86118851096031079 ) ) ;
#10846=DIRECTION ( 'NONE',  ( 0.000000000000000000, 1.000000000000000000, 0.000000000000000000 ) ) ;
#10848=VERTEX_POINT ( 'NONE', #7904 ) ;
#10861=EDGE_LOOP ( 'NONE', ( #5892, #11801 ) ) ;
#10862=DIRECTION ( 'NONE',  ( 0.000000000000000000, 1.000000000000000000, 0.000000000000000000 ) ) ;
#10864=ORIENTED_EDGE ( 'NONE', *, *, #7228, .F. ) ;
#10877=VERTEX_POINT ( 'NONE', #2177 ) ;
#10878=SURFACE_SIDE_STYLE ('',( #7937 ) ) ;
#10879=VERTEX_POINT ( 'NONE', #5807 ) ;
#10891=LINE ( 'NONE', #10013, #1213 ) ;
#10895=LINE ( 'NONE', #6159, #5242 ) ;
#10915=DIRECTION ( 'NONE',  ( 0.9595199576812789566, 0.000000000000000000, 0.2816406412635022449 ) ) ;
#10925=ORIENTED_EDGE ( 'NONE', *, *, #7034, .T. ) ;
#10928=EDGE_LOOP ( 'NONE', ( #10141, #6739, #8949, #11747 ) ) ;
#10932=CIRCLE ( 'NONE', #9954, 70.00000000000001421 ) ;
#10934=EDGE_LOOP ( 'NONE', ( #10429, #8776 ) ) ;
#10936=( LENGTH_UNIT ( ) NAMED_UNIT ( * ) SI_UNIT ( .MILLI., .METRE. ) );
#10949=PLANE ( 'NONE',  #2405 ) ;
#10951=EDGE_CURVE ( 'NONE', #3270, #1577, #5300, .T. ) ;
#10958=CARTESIAN_POINT ( 'NONE',  ( 0.000000000000000000, 52.00000000000000711, 0.000000000000000000 ) ) ;
#10959=CYLINDRICAL_SURFACE ( 'NONE', #6898, 9.999999999999994671 ) ;
#10963=EDGE_CURVE ( 'NONE', #10848, #5904, #4232, .T. ) ;
#10971=DIRECTION ( 'NONE',  ( -0.4999999999999978351, 0.000000000000000000, 0.8660254037844399289 ) ) ;
#10972=EDGE_LOOP ( 'NONE', ( #5031, #7221 ) ) ;
#10975=EDGE_CURVE ( 'NONE', #2554, #12106, #10081, .T. ) ;
#10984=CIRCLE ( 'NONE', #7201, 10.00000000000000178 ) ;
#10992=DIRECTION ( 'NONE',  ( 0.000000000000000000, 0.000000000000000000, 1.000000000000000000 ) ) ;
#10995=EDGE_LOOP ( 'NONE', ( #3489, #3400 ) ) ;
#10999=CIRCLE ( 'NONE', #5630, 70.00000000000001421 ) ;
#11019=CARTESIAN_POINT ( 'NONE',  ( 0.000000000000000000, 265.0000000000000000, 0.000000000000000000 ) ) ;
#11021=CARTESIAN_POINT ( 'NONE',  ( 1.200153863164406345E-14, 265.0000000000000000, 98.00000000000001421 ) ) ;
#11040=ORIENTED_EDGE ( 'NONE', *, *, #4104, .T. ) ;
#11042=FACE_OUTER_BOUND ( 'NONE', #1816, .T. ) ;
#11052=ORIENTED_EDGE ( 'NONE', *, *, #4179, .F. ) ;
#11058=FACE_OUTER_BOUND ( 'NONE', #3583, .T. ) ;
#11061=DIRECTION ( 'NONE',  ( 1.000000000000000000, 0.000000000000000000, 0.000000000000000000 ) ) ;
#11073=CARTESIAN_POINT ( 'NONE',  ( 24.76446302067271077, 285.0000000000000568, -102.0378428393002963 ) ) ;
#11076=VECTOR ( 'NONE', #8714, 1000.000000000000114 ) ;
#11090=LINE ( 'NONE', #11021, #7272 ) ;
#11097=DIRECTION ( 'NONE',  ( 0.000000000000000000, 1.000000000000000000, 0.000000000000000000 ) ) ;
#11098=EDGE_CURVE ( 'NONE', #1995, #3270, #3579, .T. ) ;
#11103=CARTESIAN_POINT ( 'NONE',  ( -89.80805993797480369, 275.0000000000000000, 71.82974571984181011 ) ) ;
#11104=DIRECTION ( 'NONE',  ( 0.000000000000000000, 0.000000000000000000, -1.000000000000000000 ) ) ;
#11106=CARTESIAN_POINT ( 'NONE',  ( 0.000000000000000000, 275.0000000000000000, 0.000000000000000000 ) ) ;
#11112=CARTESIAN_POINT ( 'NONE',  ( 0.000000000000000000, 265.0000000000000000, 0.000000000000000000 ) ) ;
#11124=CARTESIAN_POINT ( 'NONE',  ( 8.572527594031474570E-15, 62.00000000000000000, 70.00000000000001421 ) ) ;
#11145=CARTESIAN_POINT ( 'NONE',  ( 6.000000000000000888, 62.00000000000000000, 60.00000000000002132 ) ) ;
#11148=EDGE_CURVE ( 'NONE', #4433, #1429, #4766, .T. ) ;
#11154=EDGE_CURVE ( 'NONE', #9269, #7094, #12280, .T. ) ;
#11213=DIRECTION ( 'NONE',  ( -0.000000000000000000, -1.000000000000000000, -0.000000000000000000 ) ) ;
#11224=DIRECTION ( 'NONE',  ( 0.000000000000000000, 0.000000000000000000, 1.000000000000000000 ) ) ;
#11227=ORIENTED_EDGE ( 'NONE', *, *, #5725, .F. ) ;
#11229=FACE_OUTER_BOUND ( 'NONE', #4813, .T. ) ;
#11247=ORIENTED_EDGE ( 'NONE', *, *, #9614, .T. ) ;
#11250=DIRECTION ( 'NONE',  ( 0.000000000000000000, 0.000000000000000000, 1.000000000000000000 ) ) ;
#11252=CARTESIAN_POINT ( 'NONE',  ( 89.80805993797383735, 275.0000000000000000, 81.82974571984303225 ) ) ;
#11257=VERTEX_POINT ( 'NONE', #3921 ) ;
#11258=TOROIDAL_SURFACE ( 'NONE', #7467, 25.00000000000000000, 8.000000000000000000 ) ;
#11268=DIRECTION ( 'NONE',  ( 0.000000000000000000, 1.000000000000000000, 0.000000000000000000 ) ) ;
#11272=CARTESIAN_POINT ( 'NONE',  ( 0.000000000000000000, 115.0000000000000142, -17.00000000000000000 ) ) ;
#11274=EDGE_CURVE ( 'NONE', #8994, #10639, #1982, .T. ) ;
#11281=EDGE_CURVE ( 'NONE', #3270, #1995, #8138, .T. ) ;
#11285=CARTESIAN_POINT ( 'NONE',  ( -75.98513253586240523, 275.0000000000000000, 72.46557550663233371 ) ) ;
#11287=CARTESIAN_POINT ( 'NONE',  ( 0.000000000000000000, 260.0000000000000000, 0.000000000000000000 ) ) ;
#11301=DIRECTION ( 'NONE',  ( 0.000000000000000000, 0.000000000000000000, 1.000000000000000000 ) ) ;
#11302=LINE ( 'NONE', #5564, #223 ) ;
#11303=ORIENTED_EDGE ( 'NONE', *, *, #12194, .F. ) ;
#11318=EDGE_CURVE ( 'NONE', #6826, #4551, #991, .T. ) ;
#11325=DIRECTION ( 'NONE',  ( 0.000000000000000000, 1.000000000000000000, 0.000000000000000000 ) ) ;
#11326=CARTESIAN_POINT ( 'NONE',  ( 0.000000000000000000, 115.0000000000000142, 0.000000000000000000 ) ) ;
#11333=EDGE_LOOP ( 'NONE', ( #7371, #6759 ) ) ;
#11338=ORIENTED_EDGE ( 'NONE', *, *, #7969, .T. ) ;
#11342=AXIS2_PLACEMENT_3D ( 'NONE', #6721, #6782, #11592 ) ;
#11393=EDGE_CURVE ( 'NONE', #7317, #10706, #11740, .T. ) ;
#11396=EDGE_LOOP ( 'NONE', ( #4150, #2178, #8155, #11533 ) ) ;
#11404=ORIENTED_EDGE ( 'NONE', *, *, #9054, .F. ) ;
#11410=CARTESIAN_POINT ( 'NONE',  ( 0.000000000000000000, 50.00000000000000000, -70.00000000000001421 ) ) ;
#11459=AXIS2_PLACEMENT_3D ( 'NONE', #10476, #3056, #5744 ) ;
#11471=DIRECTION ( 'NONE',  ( 0.000000000000000000, 0.000000000000000000, -1.000000000000000000 ) ) ;
#11478=VECTOR ( 'NONE', #10622, 1000.000000000000000 ) ;
#11490=VECTOR ( 'NONE', #10731, 1000.000000000000000 ) ;
#11493=CARTESIAN_POINT ( 'NONE',  ( 0.000000000000000000, 65.00000000000000000, 0.000000000000000000 ) ) ;
#11494=EDGE_LOOP ( 'NONE', ( #7426, #6107, #6084, #8868 ) ) ;
#11497=ORIENTED_EDGE ( 'NONE', *, *, #901, .F. ) ;
#11516=EDGE_CURVE ( 'NONE', #10639, #10214, #8043, .T. ) ;
#11518=ORIENTED_EDGE ( 'NONE', *, *, #2409, .F. ) ;
#11519=VERTEX_POINT ( 'NONE', #8292 ) ;
#11521=SURFACE_STYLE_USAGE ( .BOTH. , #4913 ) ;
#11522=DIRECTION ( 'NONE',  ( 0.000000000000000000, 1.000000000000000000, 0.000000000000000000 ) ) ;
#11528=CARTESIAN_POINT ( 'NONE',  ( 89.80805993797383735, 275.0000000000000000, 71.82974571984303225 ) ) ;
#11532=EDGE_CURVE ( 'NONE', #5901, #2816, #2566, .T. ) ;
#11533=ORIENTED_EDGE ( 'NONE', *, *, #4563, .T. ) ;
#11542=SHAPE_DEFINITION_REPRESENTATION ( #9553, #3316 ) ;
#11546=ORIENTED_EDGE ( 'NONE', *, *, #8600, .F. ) ;
#11550=ORIENTED_EDGE ( 'NONE', *, *, #5332, .F. ) ;
#11554=DIRECTION ( 'NONE',  ( 0.000000000000000000, 1.000000000000000000, 0.000000000000000000 ) ) ;
#11560=VECTOR ( 'NONE', #3794, 1000.000000000000000 ) ;
#11565=AXIS2_PLACEMENT_3D ( 'NONE', #7777, #4788, #8706 ) ;
#11567=CARTESIAN_POINT ( 'NONE',  ( 0.000000000000000000, 52.00000000000000711, 0.000000000000000000 ) ) ;
#11577=AXIS2_PLACEMENT_3D ( 'NONE', #11112, #6374, #1638 ) ;
#11592=DIRECTION ( 'NONE',  ( 0.000000000000000000, 0.000000000000000000, 1.000000000000000000 ) ) ;
#11598=EDGE_CURVE ( 'NONE', #5565, #1577, #11957, .T. ) ;
#11604=CARTESIAN_POINT ( 'NONE',  ( 0.000000000000000000, 50.00000000000000000, 0.000000000000000000 ) ) ;
#11619=DIRECTION ( 'NONE',  ( 0.000000000000000000, 1.000000000000000000, 0.000000000000000000 ) ) ;
#11625=AXIS2_PLACEMENT_3D ( 'NONE', #10709, #11660, #1001 ) ;
#11646=ORIENTED_EDGE ( 'NONE', *, *, #6398, .F. ) ;
#11653=CARTESIAN_POINT ( 'NONE',  ( 6.000000000000000000, 62.00000000000000000, 70.00000000000001421 ) ) ;
#11657=AXIS2_PLACEMENT_3D ( 'NONE', #8175, #4315, #5203 ) ;
#11660=DIRECTION ( 'NONE',  ( 0.000000000000000000, 1.000000000000000000, 0.000000000000000000 ) ) ;
#11667=EDGE_CURVE ( 'NONE', #1995, #10879, #9141, .T. ) ;
#11674=DIRECTION ( 'NONE',  ( 0.000000000000000000, 0.000000000000000000, 1.000000000000000000 ) ) ;
#11681=CARTESIAN_POINT ( 'NONE',  ( 0.000000000000000000, 265.0000000000000000, 0.000000000000000000 ) ) ;
#11682=LINE ( 'NONE', #8040, #3924 ) ;
#11691=CARTESIAN_POINT ( 'NONE',  ( 0.000000000000000000, 67.00000000000000000, 0.000000000000000000 ) ) ;
#11692=EDGE_CURVE ( 'NONE', #3272, #9269, #6965, .T. ) ;
#11704=CARTESIAN_POINT ( 'NONE',  ( -116.4243635975518742, 285.0000000000000568, 45.50129185973785440 ) ) ;
#11717=DIRECTION ( 'NONE',  ( 0.000000000000000000, 1.000000000000000000, 0.000000000000000000 ) ) ;
#11729=DIRECTION ( 'NONE',  ( 0.000000000000000000, 1.000000000000000000, 0.000000000000000000 ) ) ;
#11733=CARTESIAN_POINT ( 'NONE',  ( -75.98513253586240523, 285.0000000000000568, 72.46557550663233371 ) ) ;
#11736=DIRECTION ( 'NONE',  ( 0.000000000000000000, 0.000000000000000000, 1.000000000000000000 ) ) ;
#11738=CARTESIAN_POINT ( 'NONE',  ( 0.000000000000000000, 67.00000000000000000, 0.000000000000000000 ) ) ;
#11740=LINE ( 'NONE', #4131, #8353 ) ;
#11743=AXIS2_PLACEMENT_3D ( 'NONE', #5995, #11729, #2244 ) ;
#11747=ORIENTED_EDGE ( 'NONE', *, *, #7040, .T. ) ;
#11765=EDGE_CURVE ( 'NONE', #10685, #4433, #3550, .T. ) ;
#11783=ORIENTED_EDGE ( 'NONE', *, *, #5415, .T. ) ;
#11785=EDGE_LOOP ( 'NONE', ( #9018, #5863, #7360, #3975 ) ) ;
#11786=DIRECTION ( 'NONE',  ( 0.000000000000000000, 1.000000000000000000, 0.000000000000000000 ) ) ;
#11789=CIRCLE ( 'NONE', #5015, 10.00000000000000178 ) ;
#11791=CIRCLE ( 'NONE', #6409, 17.00000000000000000 ) ;
#11796=EDGE_CURVE ( 'NONE', #2993, #6640, #9136, .T. ) ;
#11801=ORIENTED_EDGE ( 'NONE', *, *, #770, .F. ) ;
#11805=CARTESIAN_POINT ( 'NONE',  ( -100.7495955565347288, 275.0000000000000000, 29.57226733266632124 ) ) ;
#11808=ORIENTED_EDGE ( 'NONE', *, *, #9794, .T. ) ;
#11813=VERTEX_POINT ( 'NONE', #6482 ) ;
#11821=ORIENTED_EDGE ( 'NONE', *, *, #8297, .T. ) ;
#11828=AXIS2_PLACEMENT_3D ( 'NONE', #9504, #2104, #8631 ) ;
#11840=DIRECTION ( 'NONE',  ( -0.000000000000000000, -1.000000000000000000, 0.000000000000000000 ) ) ;
#11847=CARTESIAN_POINT ( 'NONE',  ( 0.000000000000000000, 285.0000000000000568, 0.000000000000000000 ) ) ;
#11867=CARTESIAN_POINT ( 'NONE',  ( 0.000000000000000000, 67.00000000000000000, -72.00000000000002842 ) ) ;
#11889=TOROIDAL_SURFACE ( 'NONE', #6516, 25.00000000000000000, 10.00000000000000000 ) ;
#11893=EDGE_CURVE ( 'NONE', #1518, #4574, #10550, .T. ) ;
#11905=DIRECTION ( 'NONE',  ( 0.000000000000000000, 0.000000000000000000, -1.000000000000000000 ) ) ;
#11926=DIRECTION ( 'NONE',  ( -0.000000000000000000, -1.000000000000000000, -0.000000000000000000 ) ) ;
#11930=DIRECTION ( 'NONE',  ( 0.000000000000000000, 0.000000000000000000, 1.000000000000000000 ) ) ;
#11936=ORIENTED_EDGE ( 'NONE', *, *, #11154, .F. ) ;
#11942=AXIS2_PLACEMENT_3D ( 'NONE', #1781, #11325, #6580 ) ;
#11951=CYLINDRICAL_SURFACE ( 'NONE', #5811, 125.0000000000000284 ) ;
#11952=DIRECTION ( 'NONE',  ( 0.9595199576812829534, 0.000000000000000000, -0.2816406412634883671 ) ) ;
#11954=DIRECTION ( 'NONE',  ( -1.224646799147352961E-16, 0.000000000000000000, 1.000000000000000000 ) ) ;
#11957=CIRCLE ( 'NONE', #3985, 9.999999999999994671 ) ;
#11961=ORIENTED_EDGE ( 'NONE', *, *, #5548, .F. ) ;
#11977=EDGE_CURVE ( 'NONE', #6060, #108, #1801, .T. ) ;
#11985=CARTESIAN_POINT ( 'NONE',  ( -107.1104145097476987, 285.0000000000000568, 41.86118851095882576 ) ) ;
#11990=LINE ( 'NONE', #5374, #1342 ) ;
#11994=VECTOR ( 'NONE', #978, 1000.000000000000000 ) ;
#11997=DIRECTION ( 'NONE',  ( 0.000000000000000000, 1.000000000000000000, 0.000000000000000000 ) ) ;
#12003=EDGE_CURVE ( 'NONE', #2376, #11519, #7893, .T. ) ;
#12008=ORIENTED_EDGE ( 'NONE', *, *, #2732, .F. ) ;
#12012=DIRECTION ( 'NONE',  ( 0.000000000000000000, 0.000000000000000000, 1.000000000000000000 ) ) ;
#12013=CARTESIAN_POINT ( 'NONE',  ( 0.000000000000000000, 275.0000000000000000, 0.000000000000000000 ) ) ;
#12017=CARTESIAN_POINT ( 'NONE',  ( -6.000000000000000000, 62.00000000000000000, 70.00000000000001421 ) ) ;
#12021=ADVANCED_FACE ( 'NONE', ( #10702 ), #8825, .F. ) ;
#12022=CARTESIAN_POINT ( 'NONE',  ( 17.30235457177317571, 275.0000000000000000, -113.6909342308024407 ) ) ;
#12029=DIRECTION ( 'NONE',  ( -0.000000000000000000, -1.000000000000000000, 0.000000000000000000 ) ) ;
#12034=ADVANCED_FACE ( 'NONE', ( #7719 ), #10584, .T. ) ;
#12036=DIRECTION ( 'NONE',  ( -0.000000000000000000, -1.000000000000000000, -0.000000000000000000 ) ) ;
#12046=ADVANCED_FACE ( 'NONE', ( #9637 ), #43, .F. ) ;
#12047=CARTESIAN_POINT ( 'NONE',  ( 9.184850993605151889E-15, 65.00000000000000000, 75.00000000000002842 ) ) ;
#12053=CYLINDRICAL_SURFACE ( 'NONE', #11577, 100.0000000000000142 ) ;
#12055=VECTOR ( 'NONE', #4868, 1000.000000000000000 ) ;
#12057=DIRECTION ( 'NONE',  ( 0.000000000000000000, 0.000000000000000000, 1.000000000000000000 ) ) ;
#12073=CIRCLE ( 'NONE', #3504, 70.00000000000001421 ) ;
#12076=AXIS2_PLACEMENT_3D ( 'NONE', #7115, #1507, #503 ) ;
#12081=DIRECTION ( 'NONE',  ( -0.8660254037844432595, 0.000000000000000000, 0.4999999999999920064 ) ) ;
#12103=EDGE_CURVE ( 'NONE', #2554, #11257, #8362, .T. ) ;
#12106=VERTEX_POINT ( 'NONE', #3355 ) ;
#12113=ORIENTED_EDGE ( 'NONE', *, *, #5036, .T. ) ;
#12124=FACE_OUTER_BOUND ( 'NONE', #4292, .T. ) ;
#12127=CARTESIAN_POINT ( 'NONE',  ( 8.572527594031474570E-15, 65.00000000000000000, 70.00000000000001421 ) ) ;
#12128=DIRECTION ( 'NONE',  ( -0.000000000000000000, -1.000000000000000000, -0.000000000000000000 ) ) ;
#12136=DIRECTION ( 'NONE',  ( 0.000000000000000000, 0.000000000000000000, -1.000000000000000000 ) ) ;
#12137=DIRECTION ( 'NONE',  ( 0.000000000000000000, 1.000000000000000000, 0.000000000000000000 ) ) ;
#12148=AXIS2_PLACEMENT_3D ( 'NONE', #3940, #7738, #6621 ) ;
#12161=AXIS2_PLACEMENT_3D ( 'NONE', #1620, #4482, #10208 ) ;
#12162=AXIS2_PLACEMENT_3D ( 'NONE', #4527, #732, #8315 ) ;
#12164=CARTESIAN_POINT ( 'NONE',  ( 0.000000000000000000, 75.00000000000001421, 25.00000000000000000 ) ) ;
#12172=PLANE ( 'NONE',  #4454 ) ;
#12178=EDGE_CURVE ( 'NONE', #8994, #4082, #10891, .T. ) ;
#12182=VECTOR ( 'NONE', #1435, 1000.000000000000000 ) ;
#12183=ORIENTED_EDGE ( 'NONE', *, *, #4193, .F. ) ;
#12189=VERTEX_POINT ( 'NONE', #2348 ) ;
#12194=EDGE_CURVE ( 'NONE', #10639, #11257, #6155, .T. ) ;
#12200=FACE_BOUND ( 'NONE', #11333, .T. ) ;
#12204=DIRECTION ( 'NONE',  ( 0.000000000000000000, 0.000000000000000000, 1.000000000000000000 ) ) ;
#12209=CIRCLE ( 'NONE', #8797, 100.0000000000000284 ) ;
#12210=DIRECTION ( 'NONE',  ( 0.000000000000000000, 1.000000000000000000, 0.000000000000000000 ) ) ;
#12213=CARTESIAN_POINT ( 'NONE',  ( -6.000000000000000000, 50.00000000000000000, 70.00000000000001421 ) ) ;
#12217=DIRECTION ( 'NONE',  ( -0.000000000000000000, -1.000000000000000000, -0.000000000000000000 ) ) ;
#12219=VERTEX_POINT ( 'NONE', #11272 ) ;
#12224=ADVANCED_FACE ( 'NONE', ( #8503 ), #7343, .T. ) ;
#12230=ORIENTED_EDGE ( 'NONE', *, *, #9433, .T. ) ;
#12245=VERTEX_POINT ( 'NONE', #5474 ) ;
#12263=DIRECTION ( 'NONE',  ( 1.000000000000000000, -0.000000000000000000, 1.224646799147353207E-16 ) ) ;
#12271=VECTOR ( 'NONE', #7260, 1000.000000000000000 ) ;
#12272=FILL_AREA_STYLE ('',( #8568 ) ) ;
#12280=LINE ( 'NONE', #3488, #2580 ) ;
#12285=ORIENTED_EDGE ( 'NONE', *, *, #7166, .T. ) ;
#12289=CIRCLE ( 'NONE', #5524, 125.0000000000000284 ) ;
#12290=DIRECTION ( 'NONE',  ( -0.000000000000000000, -1.000000000000000000, -0.000000000000000000 ) ) ;
#12300=DIRECTION ( 'NONE',  ( 0.000000000000000000, 0.000000000000000000, 1.000000000000000000 ) ) ;
#12301=ORIENTED_EDGE ( 'NONE', *, *, #6788, .T. ) ;
#12312=ORIENTED_EDGE ( 'NONE', *, *, #3308, .F. ) ;
#12317=LINE ( 'NONE', #4643, #8519 ) ;
#12325=ORIENTED_EDGE ( 'NONE', *, *, #3293, .F. ) ;
#12332=ORIENTED_EDGE ( 'NONE', *, *, #4193, .T. ) ;
#12340=CIRCLE ( 'NONE', #3174, 9.999999999999994671 ) ;
#12345=VERTEX_POINT ( 'NONE', #5537 ) ;
#12349=ORIENTED_EDGE ( 'NONE', *, *, #9179, .F. ) ;
#12350=DIRECTION ( 'NONE',  ( 0.000000000000000000, 1.000000000000000000, 0.000000000000000000 ) ) ;
#12351=VERTEX_POINT ( 'NONE', #9748 ) ;
ENDSEC;
END-ISO-10303-21;
